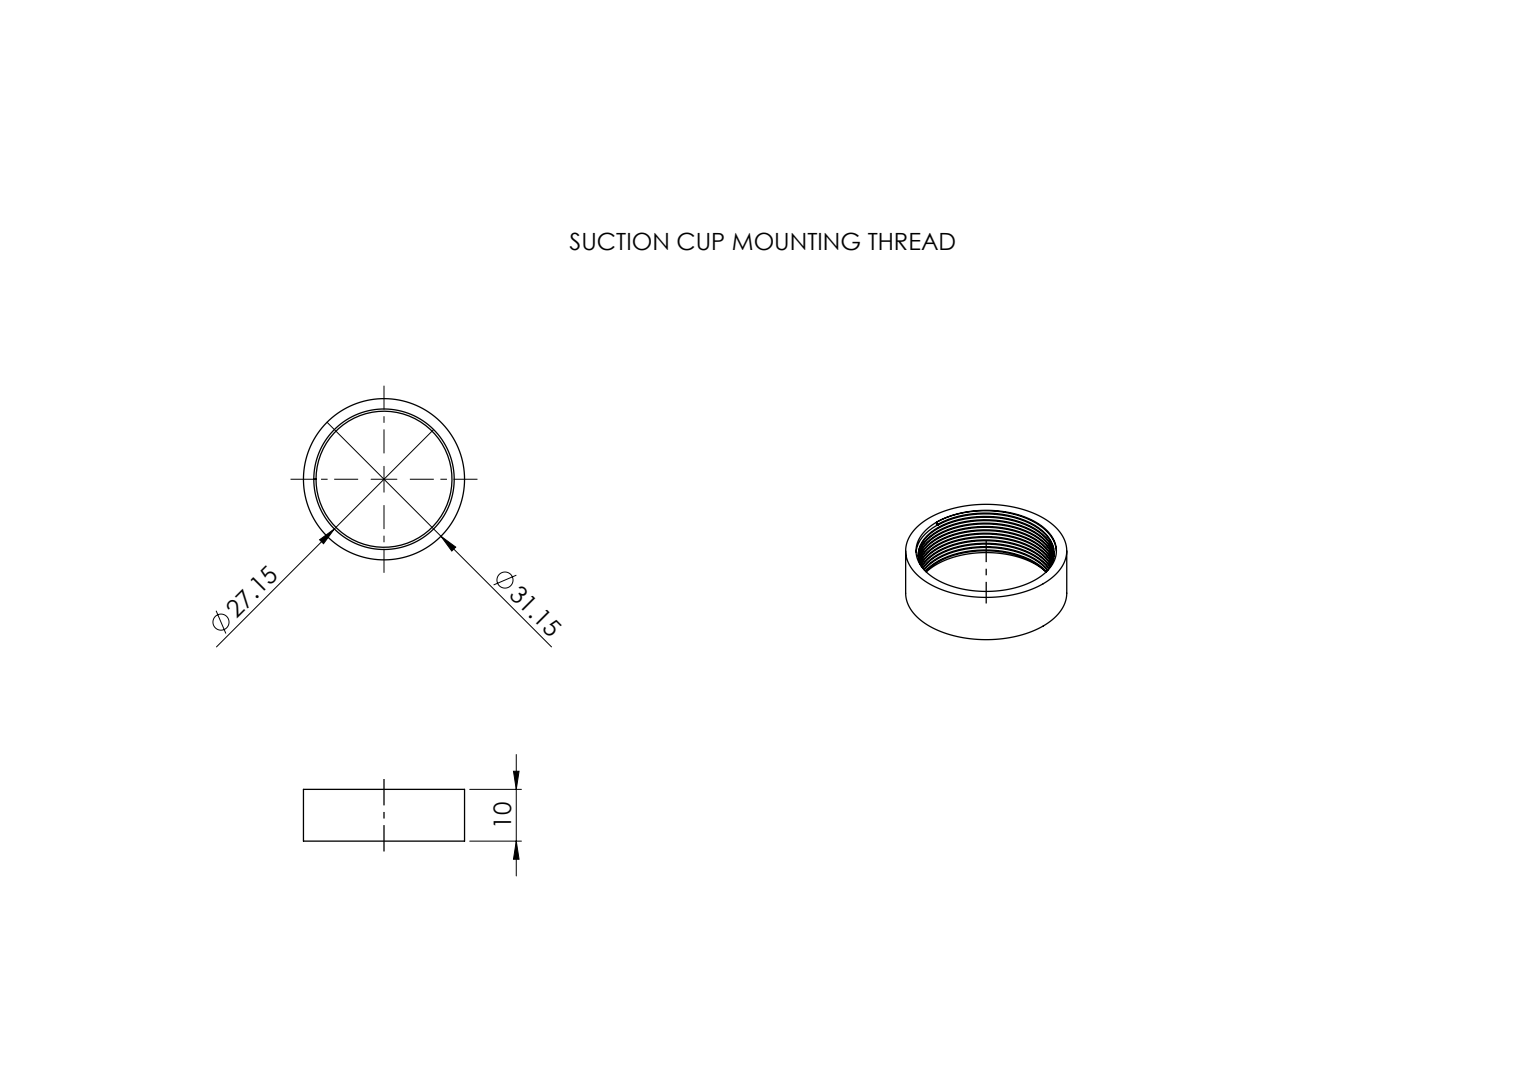
ISO-10303-21;
HEADER;
FILE_DESCRIPTION (('STEP AP214'),
    '1' );
FILE_NAME ('suction cup mounting thread.step',
    '2026-10-01T14:18:43',
    ( '' ),
    ( '' ),
    'SwSTEP 2.0',
    'SolidWorks 2026',
    '' );
FILE_SCHEMA (( 'AUTOMOTIVE_DESIGN' ));
ENDSEC;

DATA;
#15=CARTESIAN_POINT ( 'NONE',  ( 5.444914386472302859, 36.83281250108392868, 13.14518615778179189 ) ) ;
#34=VERTEX_POINT ( 'NONE', #6384 ) ;
#42=CARTESIAN_POINT ( 'NONE',  ( -13.36000105192242060, 40.87597656304196647, 0.000000000000000000 ) ) ;
#58=VERTEX_POINT ( 'NONE', #14643 ) ;
#60=CARTESIAN_POINT ( 'NONE',  ( -13.14518615778179900, 39.11484375108394573, -5.444914386472297529 ) ) ;
#65=CARTESIAN_POINT ( 'NONE',  ( -8.049105076161786076E-16, 38.96601562608393721, -13.14518615778179544 ) ) ;
#68=CARTESIAN_POINT ( 'NONE',  ( 2.493653234604083739E-15, 38.02343749999999289, 13.57481594606304576 ) ) ;
#72=CARTESIAN_POINT ( 'NONE',  ( 13.57481594606304931, 38.17226562499999432, 5.622872871577869525 ) ) ;
#73=CARTESIAN_POINT ( 'NONE',  ( 5.444914386472297529, 37.92421875108392726, -13.14518615778179900 ) ) ;
#89=CARTESIAN_POINT ( 'NONE',  ( -5.622872871577804688, 36.48554687716787726, 13.57481594606311504 ) ) ;
#92=ORIENTED_EDGE ( 'NONE', *, *, #1447, .F. ) ;
#108=CARTESIAN_POINT ( 'NONE',  ( 9.295050272127046043, 38.07304687608393579, -9.295050272127046043 ) ) ;
#109=CARTESIAN_POINT ( 'NONE',  ( -5.622872871577873077, 36.18789062716787441, -13.57481594606304753 ) ) ;
#127=CARTESIAN_POINT ( 'NONE',  ( 5.444914386472302859, 36.03906250108394005, 13.14518615778179189 ) ) ;
#138=VERTEX_POINT ( 'NONE', #3105 ) ;
#143=CARTESIAN_POINT ( 'NONE',  ( 9.598844408820456309, 34.35234374999999574, -9.598844408820458085 ) ) ;
#158=CARTESIAN_POINT ( 'NONE',  ( -9.295050272127046043, 36.48554687608393721, -9.295050272127046043 ) ) ;
#199=CARTESIAN_POINT ( 'NONE',  ( -13.14518615778179544, 37.57695312608393579, 0.000000000000000000 ) ) ;
#204=CARTESIAN_POINT ( 'NONE',  ( -9.295050272127046043, 36.68398437608393436, -9.295050272127046043 ) ) ;
#205=ADVANCED_FACE ( 'NONE', ( #10326 ), #4081, .F. ) ;
#211=CARTESIAN_POINT ( 'NONE',  ( -8.312177448680279460E-16, 36.83281249999999574, -13.57481594606304576 ) ) ;
#212=CARTESIAN_POINT ( 'NONE',  ( -13.14518615778179900, 38.12265625108393152, -5.444914386472297529 ) ) ;
#240=FACE_OUTER_BOUND ( 'NONE', #19523, .T. ) ;
#242=CARTESIAN_POINT ( 'NONE',  ( 1.662435489736055892E-15, 40.99999999999999289, 13.57481594606304576 ) ) ;
#247=CARTESIAN_POINT ( 'NONE',  ( 9.295050272127046043, 35.69179687608394147, -9.295050272127046043 ) ) ;
#248=CARTESIAN_POINT ( 'NONE',  ( 2.493653234604083739E-15, 37.32890625216786873, 13.57481594606304576 ) ) ;
#261=CARTESIAN_POINT ( 'NONE',  ( 1.662435489736055892E-15, 40.99999999999999289, 13.57481594606304576 ) ) ;
#263=ORIENTED_EDGE ( 'NONE', *, *, #18368, .T. ) ;
#269=CARTESIAN_POINT ( 'NONE',  ( -13.14518615778179189, 36.63437500108393152, 5.444914386472304635 ) ) ;
#300=CARTESIAN_POINT ( 'NONE',  ( 13.14518615778179544, 37.77539062608393294, -1.609821015232357215E-15 ) ) ;
#343=CARTESIAN_POINT ( 'NONE',  ( 2.414731522848535132E-15, 40.15664062608393436, 13.14518615778179544 ) ) ;
#349=CARTESIAN_POINT ( 'NONE',  ( 9.295050272127046043, 37.27929687608394005, -9.295050272127046043 ) ) ;
#355=CARTESIAN_POINT ( 'NONE',  ( 5.622872871577878406, 37.27929687499999289, 13.57481594606304576 ) ) ;
#356=CARTESIAN_POINT ( 'NONE',  ( -5.444914386472299306, 38.32109375108394289, 13.14518615778179722 ) ) ;
#367=PLANE ( 'NONE',  #22670 ) ;
#371=CARTESIAN_POINT ( 'NONE',  ( 0.000000000000000000, 40.99999999999999289, 0.000000000000000000 ) ) ;
#394=CARTESIAN_POINT ( 'NONE',  ( 5.444914386472297529, 38.12265625108393152, -13.14518615778179900 ) ) ;
#395=CARTESIAN_POINT ( 'NONE',  ( -9.598844408820454532, 37.22968750216787726, 9.598844408820459861 ) ) ;
#406=FACE_OUTER_BOUND ( 'NONE', #21933, .T. ) ;
#407=CARTESIAN_POINT ( 'NONE',  ( -8.312177448680279460E-16, 34.55078125216787299, -13.57481594606304576 ) ) ;
#414=CARTESIAN_POINT ( 'NONE',  ( -13.14518615778179189, 35.84062500108394289, 5.444914386472304635 ) ) ;
#416=CARTESIAN_POINT ( 'NONE',  ( 9.598844408820456309, 39.11484374999999858, -9.598844408820458085 ) ) ;
#441=CARTESIAN_POINT ( 'NONE',  ( 13.14518615778179544, 33.01289062608393010, -1.609821015232357215E-15 ) ) ;
#460=ADVANCED_FACE ( 'NONE', ( #11167, #24165 ), #367, .F. ) ;
#470=EDGE_CURVE ( 'NONE', #4431, #13527, #13159, .T. ) ;
#488=CARTESIAN_POINT ( 'NONE',  ( -9.295050272127046043, 35.09648437608393579, -9.295050272127046043 ) ) ;
#495=CARTESIAN_POINT ( 'NONE',  ( 13.14518615778179544, 36.38632812608393863, -1.609821015232357215E-15 ) ) ;
#500=CARTESIAN_POINT ( 'NONE',  ( 2.493653234604083739E-15, 33.26093749999999716, 13.57481594606304576 ) ) ;
#501=CARTESIAN_POINT ( 'NONE',  ( -8.049105076161786076E-16, 33.21132812608393436, -13.14518615778179544 ) ) ;
#535=CARTESIAN_POINT ( 'NONE',  ( -5.444914386472297529, 35.84062500108394289, -13.14518615778179900 ) ) ;
#536=CARTESIAN_POINT ( 'NONE',  ( -13.57481594606304576, 37.92421875216787441, 0.000000000000000000 ) ) ;
#548=CARTESIAN_POINT ( 'NONE',  ( -9.598844408820454532, 31.67343750216787512, 9.598844408820459861 ) ) ;
#557=CARTESIAN_POINT ( 'NONE',  ( -13.14518615778179900, 37.32890625108393579, -5.444914386472297529 ) ) ;
#586=CARTESIAN_POINT ( 'NONE',  ( -5.444914386472299306, 31.97109375108393792, 13.14518615778179722 ) ) ;
#617=AXIS2_PLACEMENT_3D ( 'NONE', #8449, #19290, #20876 ) ;
#629=CARTESIAN_POINT ( 'NONE',  ( 13.14518615778179900, 36.33671875108394289, 5.444914386472293977 ) ) ;
#636=CARTESIAN_POINT ( 'NONE',  ( -13.14518615778179189, 39.21406250108392300, 5.444914386472304635 ) ) ;
#637=VERTEX_POINT ( 'NONE', #2015 ) ;
#643=CARTESIAN_POINT ( 'NONE',  ( 5.622872871577878406, 33.31054687499999289, 13.57481594606304576 ) ) ;
#644=CARTESIAN_POINT ( 'NONE',  ( 5.444914386472297529, 33.16171875108393152, -13.14518615778179900 ) ) ;
#661=( NAMED_UNIT ( * ) SI_UNIT ( $, .STERADIAN. ) SOLID_ANGLE_UNIT ( ) );
#680=CARTESIAN_POINT ( 'NONE',  ( 13.14518615778179900, 33.95546875108393436, 5.444914386472293977 ) ) ;
#681=CARTESIAN_POINT ( 'NONE',  ( -13.57481594606304576, 33.95546875216787441, 0.000000000000000000 ) ) ;
#695=CARTESIAN_POINT ( 'NONE',  ( 0.000000000000000000, 40.99999999999999289, -13.57481594606304576 ) ) ;
#701=CARTESIAN_POINT ( 'NONE',  ( 13.14518615778179900, 34.65000000108393152, -5.444914386472297529 ) ) ;
#717=CARTESIAN_POINT ( 'NONE',  ( -8.312177448680279460E-16, 34.45156249999999432, -13.57481594606304576 ) ) ;
#729=CARTESIAN_POINT ( 'NONE',  ( -5.444914386472297529, 32.46718750108393436, -13.14518615778179722 ) ) ;
#772=CARTESIAN_POINT ( 'NONE',  ( -5.444914386472297529, 36.63437500108393152, -13.14518615778179900 ) ) ;
#779=CARTESIAN_POINT ( 'NONE',  ( -8.049105076161786076E-16, 34.99726562608393721, -13.14518615778179544 ) ) ;
#787=CARTESIAN_POINT ( 'NONE',  ( -8.312177448680279460E-16, 32.86406249999999574, -13.57481594606304576 ) ) ;
#788=CARTESIAN_POINT ( 'NONE',  ( 9.295050272127047819, 35.29492187608393294, 9.295050272127046043 ) ) ;
#797=CARTESIAN_POINT ( 'NONE',  ( 7.171391216998964424, 31.99955315621561525, -11.52591757658528948 ) ) ;
#806=SURFACE_STYLE_USAGE ( .BOTH. , #11458 ) ;
#824=ADVANCED_FACE ( 'NONE', ( #21683 ), #14677, .F. ) ;
#827=CARTESIAN_POINT ( 'NONE',  ( -5.444914386472297529, 32.66562500108393863, -13.14518615778179900 ) ) ;
#828=CARTESIAN_POINT ( 'NONE',  ( 13.57481594606304753, 35.19570312716788152, -5.622872871577873077 ) ) ;
#839=DIRECTION ( 'NONE',  ( -0.000000000000000000, -1.000000000000000000, -0.000000000000000000 ) ) ;
#846=CARTESIAN_POINT ( 'NONE',  ( -5.622872871577828668, 33.21132812499999432, 13.57481594606309194 ) ) ;
#848=CARTESIAN_POINT ( 'NONE',  ( 13.14518615778179544, 32.21914062608393436, -1.609821015232357215E-15 ) ) ;
#852=CARTESIAN_POINT ( 'NONE',  ( -8.312177448680279460E-16, 37.72578125216787726, -13.57481594606304576 ) ) ;
#859=CARTESIAN_POINT ( 'NONE',  ( -8.312177448680279460E-16, 38.51953125216787299, -13.57481594606304576 ) ) ;
#862=DIRECTION ( 'NONE',  ( -0.000000000000000000, -1.000000000000000000, -0.000000000000000000 ) ) ;
#878=CARTESIAN_POINT ( 'NONE',  ( -5.444914386472297529, 33.26093750108393721, -13.14518615778179722 ) ) ;
#891=VECTOR ( 'NONE', #4255, 1000.000000000000000 ) ;
#917=CARTESIAN_POINT ( 'NONE',  ( -8.049105076161786076E-16, 37.37851562608393863, -13.14518615778179544 ) ) ;
#924=CARTESIAN_POINT ( 'NONE',  ( -8.049105076161786076E-16, 33.40976562608393863, -13.14518615778179544 ) ) ;
#930=EDGE_CURVE ( 'NONE', #20608, #21855, #13534, .T. ) ;
#931=CARTESIAN_POINT ( 'NONE',  ( -9.598844408820458085, 32.96328124999999432, -9.598844408820458085 ) ) ;
#932=CARTESIAN_POINT ( 'NONE',  ( -8.049105076161786076E-16, 32.41757812608393863, -13.14518615778179544 ) ) ;
#937=ORIENTED_EDGE ( 'NONE', *, *, #26334, .F. ) ;
#944=CARTESIAN_POINT ( 'NONE',  ( 5.622872871578054266, 32.11992187716787583, -13.57481594606286635 ) ) ;
#947=VERTEX_POINT ( 'NONE', #24667 ) ;
#952=CYLINDRICAL_SURFACE ( 'NONE', #25355, 13.57481594606304576 ) ;
#967=CARTESIAN_POINT ( 'NONE',  ( -13.14518615778179544, 33.60820312608393579, 0.000000000000000000 ) ) ;
#968=CARTESIAN_POINT ( 'NONE',  ( 13.57481594606304753, 34.40195312716787157, -5.622872871577873077 ) ) ;
#975=CARTESIAN_POINT ( 'NONE',  ( 2.493653234604083739E-15, 37.32890625216786873, 13.57481594606304576 ) ) ;
#989=CARTESIAN_POINT ( 'NONE',  ( -13.57481594606304576, 33.06249999999999289, 0.000000000000000000 ) ) ;
#991=CARTESIAN_POINT ( 'NONE',  ( -8.049105076161786076E-16, 34.00507812608393721, -13.14518615778179544 ) ) ;
#994=CARTESIAN_POINT ( 'NONE',  ( 13.57481594606304576, 37.52734375216787299, -1.662435489736055892E-15 ) ) ;
#995=CARTESIAN_POINT ( 'NONE',  ( -13.57481594606304576, 35.44374999999999432, 0.000000000000000000 ) ) ;
#1021=CARTESIAN_POINT ( 'NONE',  ( 9.295050272127046043, 32.31835937608393294, -9.295050272127046043 ) ) ;
#1046=ORIENTED_EDGE ( 'NONE', *, *, #15737, .F. ) ;
#1060=CARTESIAN_POINT ( 'NONE',  ( 5.444914386472297529, 35.74140625108393721, -13.14518615778179900 ) ) ;
#1067=CARTESIAN_POINT ( 'NONE',  ( 9.295050272127046043, 35.69179687608394147, -9.295050272127046043 ) ) ;
#1069=CARTESIAN_POINT ( 'NONE',  ( 2.493653234604083739E-15, 36.43593749999999432, 13.57481594606304576 ) ) ;
#1072=CARTESIAN_POINT ( 'NONE',  ( -13.57481594606304576, 32.26874999999999716, 0.000000000000000000 ) ) ;
#1073=CARTESIAN_POINT ( 'NONE',  ( 13.14518615778179900, 34.65000000108393152, -5.444914386472297529 ) ) ;
#1109=CARTESIAN_POINT ( 'NONE',  ( -9.295050272127046043, 33.50898437608393010, -9.295050272127046043 ) ) ;
#1110=CARTESIAN_POINT ( 'NONE',  ( 2.493653234604083739E-15, 35.74140625216787015, 13.57481594606304576 ) ) ;
#1119=EDGE_LOOP ( 'NONE', ( #16453, #20874 ) ) ;
#1129=CARTESIAN_POINT ( 'NONE',  ( 13.57481594606304753, 40.65273437499999432, -5.622872871577873966 ) ) ;
#1131=CARTESIAN_POINT ( 'NONE',  ( 13.14518615778179544, 33.80664062608393294, -1.609821015232357215E-15 ) ) ;
#1135=CARTESIAN_POINT ( 'NONE',  ( 5.622872871577786924, 37.37851562716787157, 13.57481594606313813 ) ) ;
#1171=CARTESIAN_POINT ( 'NONE',  ( 9.598844408820459861, 35.84062500216786873, 9.598844408820456309 ) ) ;
#1201=CARTESIAN_POINT ( 'NONE',  ( 9.295050272127046043, 33.31054687608394005, -9.295050272127046043 ) ) ;
#1209=CARTESIAN_POINT ( 'NONE',  ( 2.414731522848535132E-15, 36.18789062608393436, 13.14518615778179544 ) ) ;
#1225=CARTESIAN_POINT ( 'NONE',  ( -5.622872871577873966, 33.70742187499999432, -13.57481594606304753 ) ) ;
#1231=ORIENTED_EDGE ( 'NONE', *, *, #22053, .F. ) ;
#1245=CARTESIAN_POINT ( 'NONE',  ( 2.414731522848535132E-15, 32.21914062608393436, 13.14518615778179544 ) ) ;
#1246=CARTESIAN_POINT ( 'NONE',  ( -5.622872871577873077, 33.31054687716787299, 13.57481594606304753 ) ) ;
#1265=LINE ( 'NONE', #3115, #23908 ) ;
#1267=CARTESIAN_POINT ( 'NONE',  ( -13.14518615778179544, 34.20351562608393436, 0.000000000000000000 ) ) ;
#1308=CARTESIAN_POINT ( 'NONE',  ( 0.000000000000000000, 40.99999999999999289, 0.000000000000000000 ) ) ;
#1310=AXIS2_PLACEMENT_3D ( 'NONE', #21064, #21343, #23065 ) ;
#1313=EDGE_CURVE ( 'NONE', #21025, #17571, #11932, .T. ) ;
#1317=ORIENTED_EDGE ( 'NONE', *, *, #20419, .T. ) ;
#1326=CARTESIAN_POINT ( 'NONE',  ( -5.444914386472297529, 39.61093750108393152, -13.14518615778179722 ) ) ;
#1337=CARTESIAN_POINT ( 'NONE',  ( 6.944426393311538881, 31.75150625057403175, -11.16113171639042356 ) ) ;
#1344=CARTESIAN_POINT ( 'NONE',  ( -5.444914386472297529, 35.04687500108393294, -13.14518615778179722 ) ) ;
#1355=ORIENTED_EDGE ( 'NONE', *, *, #12984, .F. ) ;
#1377=DIRECTION ( 'NONE',  ( 0.000000000000000000, 1.000000000000000000, 0.000000000000000000 ) ) ;
#1385=CARTESIAN_POINT ( 'NONE',  ( -13.57481594606304753, 40.15664062500000142, -5.622872871577873077 ) ) ;
#1386=CARTESIAN_POINT ( 'NONE',  ( -13.57481594606304753, 32.31835937716786589, -5.622872871577873077 ) ) ;
#1403=CARTESIAN_POINT ( 'NONE',  ( 0.000000000000000000, 40.99999999999999289, -13.57481594606304576 ) ) ;
#1406=EDGE_LOOP ( 'NONE', ( #23949, #8331, #11999, #3725 ) ) ;
#1447=EDGE_CURVE ( 'NONE', #17326, #28027, #2482, .T. ) ;
#1466=CARTESIAN_POINT ( 'NONE',  ( -5.444914386472297529, 38.02343750108394005, -13.14518615778179722 ) ) ;
#1474=CARTESIAN_POINT ( 'NONE',  ( 2.414731522848535132E-15, 33.80664062608393294, 13.14518615778179544 ) ) ;
#1494=VERTEX_POINT ( 'NONE', #14891 ) ;
#1503=DIRECTION ( 'NONE',  ( -0.8490667072653959035, 1.618318251311064231E-06, -0.5282856486891157610 ) ) ;
#1513=CARTESIAN_POINT ( 'NONE',  ( 9.295050272127047819, 40.25585937608393294, 9.295050272127046043 ) ) ;
#1519=AXIS2_PLACEMENT_3D ( 'NONE', #14564, #16851, #14693 ) ;
#1522=CARTESIAN_POINT ( 'NONE',  ( 5.622872871577871301, 38.37070312499999147, -13.57481594606304753 ) ) ;
#1523=CARTESIAN_POINT ( 'NONE',  ( 2.493653234604083739E-15, 32.56640625216787299, 13.57481594606304576 ) ) ;
#1532=FACE_OUTER_BOUND ( 'NONE', #20108, .T. ) ;
#1541=AXIS2_PLACEMENT_3D ( 'NONE', #2821, #839, #9509 ) ;
#1564=CARTESIAN_POINT ( 'NONE',  ( 9.295050272127046043, 39.66054687608393436, -9.295050272127046043 ) ) ;
#1605=CARTESIAN_POINT ( 'NONE',  ( 9.295050272127046043, 37.87460937608393152, -9.295050272127046043 ) ) ;
#1609=ORIENTED_EDGE ( 'NONE', *, *, #12107, .F. ) ;
#1614=CARTESIAN_POINT ( 'NONE',  ( 9.295050272127046043, 34.10429687608393579, -9.295050272127046043 ) ) ;
#1621=CARTESIAN_POINT ( 'NONE',  ( 13.14518615778179544, 32.41757812608393863, -1.609821015232357215E-15 ) ) ;
#1627=CARTESIAN_POINT ( 'NONE',  ( -5.622872871577965448, 32.41757812499999858, 13.57481594606295161 ) ) ;
#1640=CARTESIAN_POINT ( 'NONE',  ( 9.598844408820459861, 31.87187500216787228, 9.598844408820456309 ) ) ;
#1654=CARTESIAN_POINT ( 'NONE',  ( 5.622872871577878406, 39.66054687500000142, 13.57481594606304576 ) ) ;
#1655=CARTESIAN_POINT ( 'NONE',  ( -5.444914386472297529, 40.40468750108393436, -13.14518615778179900 ) ) ;
#1690=APPLICATION_CONTEXT ( 'automotive_design' ) ;
#1698=CARTESIAN_POINT ( 'NONE',  ( 13.14518615778179900, 40.40468750108393436, -5.444914386472297529 ) ) ;
#1716=CARTESIAN_POINT ( 'NONE',  ( -5.444914386472299306, 39.11484375108394573, 13.14518615778179722 ) ) ;
#1722=DIRECTION ( 'NONE',  ( 1.374060148949977908E-06, 0.9999999999986906030, 8.549343071804204525E-07 ) ) ;
#1734=ORIENTED_EDGE ( 'NONE', *, *, #1871, .F. ) ;
#1742=CARTESIAN_POINT ( 'NONE',  ( -5.444914386472297529, 38.81718750108393579, -13.14518615778179722 ) ) ;
#1753=CARTESIAN_POINT ( 'NONE',  ( 13.14518615778179544, 32.41757812608393863, -1.609821015232357215E-15 ) ) ;
#1783=CARTESIAN_POINT ( 'NONE',  ( -8.049105076161786076E-16, 33.21132812608393436, -13.14518615778179544 ) ) ;
#1796=CARTESIAN_POINT ( 'NONE',  ( -13.57481594606304753, 40.95039062499999005, -5.622872871577873077 ) ) ;
#1797=CARTESIAN_POINT ( 'NONE',  ( 5.444914386472302859, 39.21406250108392300, 13.14518615778179189 ) ) ;
#1809=CARTESIAN_POINT ( 'NONE',  ( -5.622872871577873966, 34.79882812499999289, 13.57481594606304753 ) ) ;
#1816=ORIENTED_EDGE ( 'NONE', *, *, #14513, .T. ) ;
#1838=CARTESIAN_POINT ( 'NONE',  ( -9.598844408820458085, 40.20625000216787726, -9.598844408820458085 ) ) ;
#1854=CARTESIAN_POINT ( 'NONE',  ( -5.444914386472297529, 38.02343750108394005, -13.14518615778179900 ) ) ;
#1871=EDGE_CURVE ( 'NONE', #9928, #16597, #27628, .T. ) ;
#1876=CARTESIAN_POINT ( 'NONE',  ( -13.57481594606304398, 33.21132812716787441, 5.622872871577880183 ) ) ;
#1879=ORIENTED_EDGE ( 'NONE', *, *, #9511, .T. ) ;
#1883=CARTESIAN_POINT ( 'NONE',  ( 5.444914386472302859, 39.21406250108392300, 13.14518615778179189 ) ) ;
#1906=CARTESIAN_POINT ( 'NONE',  ( -13.57481594606304576, 37.13046875216787868, 0.000000000000000000 ) ) ;
#1911=DIRECTION ( 'NONE',  ( 1.000000000000000000, 0.000000000000000000, -0.000000000000000000 ) ) ;
#1912=CARTESIAN_POINT ( 'NONE',  ( 0.000000000000000000, 40.99999999999999289, 0.000000000000000000 ) ) ;
#1919=CYLINDRICAL_SURFACE ( 'NONE', #9601, 13.57481594606304576 ) ;
#1923=CARTESIAN_POINT ( 'NONE',  ( 5.444914386472302859, 38.61875000108393152, 13.14518615778179189 ) ) ;
#1928=CARTESIAN_POINT ( 'NONE',  ( 2.414731522848535132E-15, 40.15664062608393436, 13.14518615778179544 ) ) ;
#1934=CARTESIAN_POINT ( 'NONE',  ( -5.622872871577873077, 39.26367187499999289, -13.57481594606304753 ) ) ;
#1935=CARTESIAN_POINT ( 'NONE',  ( 5.444914386472297529, 40.30546875108393579, -13.14518615778179900 ) ) ;
#1949=( LENGTH_UNIT ( ) NAMED_UNIT ( * ) SI_UNIT ( .MILLI., .METRE. ) );
#1968=ORIENTED_EDGE ( 'NONE', *, *, #8452, .F. ) ;
#1970=CARTESIAN_POINT ( 'NONE',  ( 13.14518615778179900, 38.81718750108393579, -5.444914386472297529 ) ) ;
#1989=CARTESIAN_POINT ( 'NONE',  ( -13.14518615778179900, 38.12265625108393152, -5.444914386472297529 ) ) ;
#2000=VERTEX_POINT ( 'NONE', #4164 ) ;
#2006=EDGE_LOOP ( 'NONE', ( #20300, #6817, #20484, #23254 ) ) ;
#2014=CARTESIAN_POINT ( 'NONE',  ( 13.14518615778179544, 36.18789062608393436, -1.609821015232357215E-15 ) ) ;
#2015=CARTESIAN_POINT ( 'NONE',  ( 1.662435489736055892E-15, 40.99999999999999289, 13.57481594606304576 ) ) ;
#2021=DIRECTION ( 'NONE',  ( -0.000000000000000000, -1.000000000000000000, -0.000000000000000000 ) ) ;
#2029=CARTESIAN_POINT ( 'NONE',  ( 1.662435489736055892E-15, 40.99999999999999289, 13.57481594606304576 ) ) ;
#2058=CARTESIAN_POINT ( 'NONE',  ( 9.295050272127046043, 38.07304687608393579, -9.295050272127046043 ) ) ;
#2063=CARTESIAN_POINT ( 'NONE',  ( 13.14518615778179722, 40.40468750108393436, -5.444914386472297529 ) ) ;
#2065=CARTESIAN_POINT ( 'NONE',  ( -13.57481594606304753, 37.77539062499998579, -5.622872871577872189 ) ) ;
#2069=CARTESIAN_POINT ( 'NONE',  ( -5.622872871577873077, 36.88242187499999858, -13.57481594606304753 ) ) ;
#2070=CARTESIAN_POINT ( 'NONE',  ( -5.444914386472299306, 35.93984375108392726, 13.14518615778179722 ) ) ;
#2077=ORIENTED_EDGE ( 'NONE', *, *, #19944, .F. ) ;
#2089=VECTOR ( 'NONE', #21736, 1000.000000000000000 ) ;
#2101=CARTESIAN_POINT ( 'NONE',  ( -13.57481594606304753, 39.36289062499999858, -5.622872871577872189 ) ) ;
#2102=CARTESIAN_POINT ( 'NONE',  ( -8.312177448680279460E-16, 37.62656249999999858, -13.57481594606304576 ) ) ;
#2108=CARTESIAN_POINT ( 'NONE',  ( -13.14518615778179544, 38.37070312608393152, 0.000000000000000000 ) ) ;
#2109=CARTESIAN_POINT ( 'NONE',  ( -13.57481594606304753, 36.28710937716787299, -5.622872871577873077 ) ) ;
#2116=VERTEX_POINT ( 'NONE', #21973 ) ;
#2128=CARTESIAN_POINT ( 'NONE',  ( 9.295050272127047819, 40.05742187608392868, 9.295050272127046043 ) ) ;
#2157=( BOUNDED_CURVE ( )  B_SPLINE_CURVE ( 2, ( #26013, #4216, #6076, #14743, #12873, #4080, #6345, #13012, #10612 ),
 .UNSPECIFIED., .F., .F. ) 
 B_SPLINE_CURVE_WITH_KNOTS ( ( 3, 2, 2, 2, 3 ),
 ( 0.1458333333333336757, 0.1562500000000002776, 0.1666666666666669072, 0.1770833333333335369, 0.1875000000000001388 ),
 .UNSPECIFIED. ) 
 CURVE ( )  GEOMETRIC_REPRESENTATION_ITEM ( )  RATIONAL_B_SPLINE_CURVE ( ( 0.9999999999999975575, 0.9238795325112891810, 1.000000000000000000, 0.9238795325112867385, 1.000000000000000000, 0.9238795325112867385, 1.000000000000000000, 0.9238795325112857393, 1.000000000000001110 ) ) 
 REPRESENTATION_ITEM ( '' )  );
#2158=CARTESIAN_POINT ( 'NONE',  ( 13.14518615778179722, 35.34453125108392157, 5.444914386472293977 ) ) ;
#2164=FACE_OUTER_BOUND ( 'NONE', #18756, .T. ) ;
#2202=CARTESIAN_POINT ( 'NONE',  ( -8.049105076161786076E-16, 40.55351562608393579, -13.14518615778179544 ) ) ;
#2208=CARTESIAN_POINT ( 'NONE',  ( 13.14518615778179722, 39.51171875108393294, 5.444914386472293977 ) ) ;
#2209=CARTESIAN_POINT ( 'NONE',  ( -5.622872871577890841, 39.66054687716787441, 13.57481594606302444 ) ) ;
#2213=AXIS2_PLACEMENT_3D ( 'NONE', #10774, #17198, #4241 ) ;
#2216=CARTESIAN_POINT ( 'NONE',  ( -13.57481594606304576, 37.03124999999999289, 0.000000000000000000 ) ) ;
#2217=CARTESIAN_POINT ( 'NONE',  ( -13.14518615778179189, 35.84062500108394289, 5.444914386472304635 ) ) ;
#2231=CARTESIAN_POINT ( 'NONE',  ( -9.598844408820454532, 34.74921874999999716, 9.598844408820459861 ) ) ;
#2233=VECTOR ( 'NONE', #26227, 1000.000000000000000 ) ;
#2247=B_SPLINE_CURVE_WITH_KNOTS ( 'NONE', 3,
 ( #26875, #18454, #5344, #2915 ),
 .UNSPECIFIED., .F., .F.,
 ( 4, 4 ),
 ( 0.000000000000000000, 1.000000000000000000 ),
 .UNSPECIFIED. ) ;
#2248=CYLINDRICAL_SURFACE ( 'NONE', #9842, 13.57481594606304576 ) ;
#2250=DIRECTION ( 'NONE',  ( -0.000000000000000000, -1.000000000000000000, -0.000000000000000000 ) ) ;
#2254=CARTESIAN_POINT ( 'NONE',  ( -8.312177448680279460E-16, 34.55078125216787299, -13.57481594606304576 ) ) ;
#2255=CARTESIAN_POINT ( 'NONE',  ( -13.14518615778179544, 37.57695312608393579, 0.000000000000000000 ) ) ;
#2256=CARTESIAN_POINT ( 'NONE',  ( -5.622872871577873077, 37.27929687716787299, 13.57481594606304753 ) ) ;
#2273=CARTESIAN_POINT ( 'NONE',  ( 0.000000000000000000, 40.99999999999999289, -15.57481594606304576 ) ) ;
#2275=CARTESIAN_POINT ( 'NONE',  ( 2.414731522848535132E-15, 39.16445312608392726, 13.14518615778179544 ) ) ;
#2278=DIRECTION ( 'NONE',  ( 0.000000000000000000, 0.000000000000000000, -1.000000000000000000 ) ) ;
#2291=CARTESIAN_POINT ( 'NONE',  ( 13.57481594606304931, 34.20351562499999432, 5.622872871577868636 ) ) ;
#2302=CARTESIAN_POINT ( 'NONE',  ( 5.444914386472297529, 37.13046875108393152, -13.14518615778179722 ) ) ;
#2311=CARTESIAN_POINT ( 'NONE',  ( 0.000000000000000000, 40.99999999999999289, 0.000000000000000000 ) ) ;
#2315=LINE ( 'NONE', #15103, #16400 ) ;
#2316=DIRECTION ( 'NONE',  ( -0.000000000000000000, -1.000000000000000000, -0.000000000000000000 ) ) ;
#2317=FACE_OUTER_BOUND ( 'NONE', #13417, .T. ) ;
#2339=CARTESIAN_POINT ( 'NONE',  ( 0.000000000000000000, 40.99999999999999289, 0.000000000000000000 ) ) ;
#2345=CARTESIAN_POINT ( 'NONE',  ( -13.14518615778179900, 38.32109375108394289, -5.444914386472297529 ) ) ;
#2351=CARTESIAN_POINT ( 'NONE',  ( -9.295050272127044266, 38.46992187608393721, 9.295050272127047819 ) ) ;
#2358=CARTESIAN_POINT ( 'NONE',  ( -9.598844408820458085, 35.34453124999998863, -9.598844408820458085 ) ) ;
#2359=CARTESIAN_POINT ( 'NONE',  ( 5.444914386472302859, 36.03906250108394005, 13.14518615778179189 ) ) ;
#2372=CARTESIAN_POINT ( 'NONE',  ( -9.598844408820458085, 34.55078124999999289, -9.598844408820458085 ) ) ;
#2373=EDGE_CURVE ( 'NONE', #2719, #1494, #18964, .T. ) ;
#2396=CARTESIAN_POINT ( 'NONE',  ( -9.295050272127046043, 38.27148437608393294, -9.295050272127046043 ) ) ;
#2397=CARTESIAN_POINT ( 'NONE',  ( -8.312177448680279460E-16, 38.51953125216787299, -13.57481594606304576 ) ) ;
#2416=CARTESIAN_POINT ( 'NONE',  ( -5.444914386472299306, 35.14609375108393152, 13.14518615778179722 ) ) ;
#2442=CARTESIAN_POINT ( 'NONE',  ( 9.295050272127046043, 37.08085937608393579, -9.295050272127046043 ) ) ;
#2460=CARTESIAN_POINT ( 'NONE',  ( 0.000000000000000000, 40.99999999999999289, -13.57481594606304576 ) ) ;
#2469=CARTESIAN_POINT ( 'NONE',  ( 13.57481594606304576, 33.55859375216787299, -1.662435489736055892E-15 ) ) ;
#2475=CARTESIAN_POINT ( 'NONE',  ( 13.57481594606304576, 37.42812499999999432, -1.662435489736055892E-15 ) ) ;
#2479=CARTESIAN_POINT ( 'NONE',  ( -5.444914386472297529, 39.80937500108392868, -13.14518615778179900 ) ) ;
#2482=( BOUNDED_CURVE ( )  B_SPLINE_CURVE ( 2, ( #20922, #23059, #27618, #3809, #6224, #16771, #25328, #12469, #10336 ),
 .UNSPECIFIED., .F., .F. ) 
 B_SPLINE_CURVE_WITH_KNOTS ( ( 3, 2, 2, 2, 3 ),
 ( 0.8124999999999998890, 0.8229166666666666297, 0.8333333333333334814, 0.8437500000000003331, 0.8541666666666670737 ),
 .UNSPECIFIED. ) 
 CURVE ( )  GEOMETRIC_REPRESENTATION_ITEM ( )  RATIONAL_B_SPLINE_CURVE ( ( 1.000000000000000888, 0.9238795325112859613, 1.000000000000000000, 0.9238795325112867385, 1.000000000000000000, 0.9238795325112867385, 1.000000000000000000, 0.9238795325112835188, 1.000000000000003331 ) ) 
 REPRESENTATION_ITEM ( '' )  );
#2486=CARTESIAN_POINT ( 'NONE',  ( -13.14518615778179722, 38.32109375108394289, -5.444914386472297529 ) ) ;
#2493=CARTESIAN_POINT ( 'NONE',  ( -5.622872871577873077, 36.08867187500000284, -13.57481594606304753 ) ) ;
#2494=CARTESIAN_POINT ( 'NONE',  ( -8.049105076161786076E-16, 35.59257812608393579, -13.14518615778179544 ) ) ;
#2508=CARTESIAN_POINT ( 'NONE',  ( -13.57481594606304398, 36.38632812716788578, 5.622872871577880183 ) ) ;
#2517=DIRECTION ( 'NONE',  ( 0.000000000000000000, 1.000000000000000000, 0.000000000000000000 ) ) ;
#2523=CARTESIAN_POINT ( 'NONE',  ( -8.312177448680279460E-16, 39.21406249999999716, -13.57481594606304576 ) ) ;
#2530=CARTESIAN_POINT ( 'NONE',  ( -13.14518615778179189, 36.03906250108394005, 5.444914386472304635 ) ) ;
#2531=CARTESIAN_POINT ( 'NONE',  ( -5.622872871577873077, 37.77539062716788010, -13.57481594606304753 ) ) ;
#2548=CARTESIAN_POINT ( 'NONE',  ( 13.57481594606304576, 34.35234375216787583, -1.662435489736055892E-15 ) ) ;
#2553=DIRECTION ( 'NONE',  ( -0.000000000000000000, -1.000000000000000000, -0.000000000000000000 ) ) ;
#2555=CARTESIAN_POINT ( 'NONE',  ( 9.295050272127047819, 37.67617187608393436, 9.295050272127046043 ) ) ;
#2585=CARTESIAN_POINT ( 'NONE',  ( 5.444914386472297529, 35.54296875108393294, -13.14518615778179722 ) ) ;
#2607=ORIENTED_EDGE ( 'NONE', *, *, #18989, .F. ) ;
#2625=CARTESIAN_POINT ( 'NONE',  ( -13.14518615778179544, 35.19570312608393436, 0.000000000000000000 ) ) ;
#2632=CARTESIAN_POINT ( 'NONE',  ( 5.444914386472297529, 38.91640625108393436, -13.14518615778179722 ) ) ;
#2637=CARTESIAN_POINT ( 'NONE',  ( 13.57481594606304931, 37.37851562499999858, 5.622872871577869525 ) ) ;
#2638=CARTESIAN_POINT ( 'NONE',  ( 13.14518615778179900, 36.93203125108394147, 5.444914386472293977 ) ) ;
#2674=CARTESIAN_POINT ( 'NONE',  ( 13.14518615778179900, 37.22968750108393721, -5.444914386472297529 ) ) ;
#2675=CARTESIAN_POINT ( 'NONE',  ( 9.598844408820456309, 38.42031250216787441, -9.598844408820458085 ) ) ;
#2681=VECTOR ( 'NONE', #18208, 1000.000000000000000 ) ;
#2695=CARTESIAN_POINT ( 'NONE',  ( -8.049105076161786076E-16, 35.59257812608393579, -13.14518615778179544 ) ) ;
#2719=VERTEX_POINT ( 'NONE', #7023 ) ;
#2725=CARTESIAN_POINT ( 'NONE',  ( 13.14518615778179544, 34.60039062608392868, -1.609821015232357215E-15 ) ) ;
#2742=ORIENTED_EDGE ( 'NONE', *, *, #930, .F. ) ;
#2766=CARTESIAN_POINT ( 'NONE',  ( -9.295050272127046043, 35.89023437608393152, -9.295050272127046043 ) ) ;
#2772=CARTESIAN_POINT ( 'NONE',  ( -5.444914386472299306, 38.51953125108393294, 13.14518615778179722 ) ) ;
#2773=CARTESIAN_POINT ( 'NONE',  ( -8.312177448680279460E-16, 36.03906250000000000, -13.57481594606304576 ) ) ;
#2777=CARTESIAN_POINT ( 'NONE',  ( -9.598844408820458085, 32.16953124999999147, -9.598844408820458085 ) ) ;
#2778=CARTESIAN_POINT ( 'NONE',  ( -9.295050272127046043, 34.89804687608393152, -9.295050272127046043 ) ) ;
#2784=ORIENTED_EDGE ( 'NONE', *, *, #12107, .T. ) ;
#2790=CARTESIAN_POINT ( 'NONE',  ( 2.493653234604083739E-15, 36.43593749999999432, 13.57481594606304576 ) ) ;
#2809=CARTESIAN_POINT ( 'NONE',  ( -5.444914386472299306, 32.16953125108393152, 13.14518615778179722 ) ) ;
#2810=CARTESIAN_POINT ( 'NONE',  ( 9.598844408820456309, 35.24531250216787726, -9.598844408820458085 ) ) ;
#2821=CARTESIAN_POINT ( 'NONE',  ( 0.000000000000000000, 40.99999999999999289, 0.000000000000000000 ) ) ;
#2831=CARTESIAN_POINT ( 'NONE',  ( 9.295050272127046043, 34.69960937608393436, -9.295050272127046043 ) ) ;
#2834=CARTESIAN_POINT ( 'NONE',  ( -5.622872871577839327, 38.07304687716787583, 13.57481594606308128 ) ) ;
#2847=CARTESIAN_POINT ( 'NONE',  ( 9.598844408820459861, 34.15390624999999858, 9.598844408820456309 ) ) ;
#2858=CARTESIAN_POINT ( 'NONE',  ( -5.444914386472299306, 33.55859375108393294, 13.14518615778179722 ) ) ;
#2899=CARTESIAN_POINT ( 'NONE',  ( -13.14518615778179900, 36.73359375108393010, -5.444914386472297529 ) ) ;
#2905=CARTESIAN_POINT ( 'NONE',  ( 5.444914386472302859, 35.44375000108393436, 13.14518615778179189 ) ) ;
#2911=CARTESIAN_POINT ( 'NONE',  ( -5.622872871577873077, 34.79882812499998579, 13.57481594606304753 ) ) ;
#2912=CARTESIAN_POINT ( 'NONE',  ( -13.14518615778179544, 34.20351562608393436, 0.000000000000000000 ) ) ;
#2915=CARTESIAN_POINT ( 'NONE',  ( 7.171390501253594785, 31.30502191632583830, -11.52591802191987114 ) ) ;
#2917=EDGE_LOOP ( 'NONE', ( #4462, #19296, #4936, #14694 ) ) ;
#2924=CARTESIAN_POINT ( 'NONE',  ( -13.57481594606304753, 34.69960937716787441, -5.622872871577872189 ) ) ;
#2942=EDGE_LOOP ( 'NONE', ( #20773, #11386, #17741, #16971 ) ) ;
#2945=CARTESIAN_POINT ( 'NONE',  ( -5.444914386472299306, 34.55078125108393294, 13.14518615778179722 ) ) ;
#2946=CARTESIAN_POINT ( 'NONE',  ( -9.598844408820458085, 33.06250000216787299, -9.598844408820458085 ) ) ;
#2965=CARTESIAN_POINT ( 'NONE',  ( -13.14518615778179900, 36.53515625108392584, -5.444914386472297529 ) ) ;
#2998=CARTESIAN_POINT ( 'NONE',  ( -5.444914386472297529, 34.05468750108393294, -13.14518615778179722 ) ) ;
#3008=CARTESIAN_POINT ( 'NONE',  ( 0.000000000000000000, 30.99999999999999645, 0.000000000000000000 ) ) ;
#3019=CARTESIAN_POINT ( 'NONE',  ( 13.57481594606304753, 39.95820312716787726, -5.622872871577873966 ) ) ;
#3041=CARTESIAN_POINT ( 'NONE',  ( 2.414731522848535132E-15, 36.98164062608393721, 13.14518615778179544 ) ) ;
#3049=CARTESIAN_POINT ( 'NONE',  ( 9.295050272127047819, 34.69960937608393436, 9.295050272127046043 ) ) ;
#3057=CARTESIAN_POINT ( 'NONE',  ( -9.598844408820454532, 33.16171874999999858, 9.598844408820459861 ) ) ;
#3058=CARTESIAN_POINT ( 'NONE',  ( -13.14518615778179544, 32.61601562608393579, 0.000000000000000000 ) ) ;
#3073=CARTESIAN_POINT ( 'NONE',  ( -8.312177448680279460E-16, 32.16953125216787157, -13.57481594606304576 ) ) ;
#3077=PRESENTATION_STYLE_ASSIGNMENT (( #806 ) ) ;
#3093=ORIENTED_EDGE ( 'NONE', *, *, #13327, .F. ) ;
#3095=CARTESIAN_POINT ( 'NONE',  ( -5.444914386472297529, 33.45937500108394147, -13.14518615778179900 ) ) ;
#3096=CARTESIAN_POINT ( 'NONE',  ( -5.622872871577873077, 34.60039062716786873, -13.57481594606304753 ) ) ;
#3105=CARTESIAN_POINT ( 'NONE',  ( 2.493653234604083739E-15, 38.91640625216786731, 13.57481594606304576 ) ) ;
#3107=CARTESIAN_POINT ( 'NONE',  ( -8.312177448680279460E-16, 31.37578125216787583, -13.57481594606304576 ) ) ;
#3115=CARTESIAN_POINT ( 'NONE',  ( 1.662435489736055892E-15, 40.99999999999999289, 13.57481594606304576 ) ) ;
#3117=CARTESIAN_POINT ( 'NONE',  ( -5.444914386472299306, 33.55859375108393294, 13.14518615778179722 ) ) ;
#3121=CARTESIAN_POINT ( 'NONE',  ( -8.312177448680279460E-16, 37.72578125216787726, -13.57481594606304576 ) ) ;
#3149=CARTESIAN_POINT ( 'NONE',  ( -8.049105076161786076E-16, 32.41757812608393863, -13.14518615778179544 ) ) ;
#3154=CARTESIAN_POINT ( 'NONE',  ( 5.622872871578008080, 36.08867187716787583, -13.57481594606290898 ) ) ;
#3185=CARTESIAN_POINT ( 'NONE',  ( -5.444914386472299306, 35.34453125108393579, 13.14518615778179722 ) ) ;
#3190=CARTESIAN_POINT ( 'NONE',  ( 13.14518615778179722, 35.54296875108394715, 5.444914386472293977 ) ) ;
#3196=CARTESIAN_POINT ( 'NONE',  ( 5.622872871577878406, 34.10429687499999574, 13.57481594606304576 ) ) ;
#3197=CARTESIAN_POINT ( 'NONE',  ( -5.444914386472297529, 34.84843750108393579, -13.14518615778179900 ) ) ;
#3209=ADVANCED_FACE ( 'NONE', ( #19413 ), #19987, .F. ) ;
#3211=CARTESIAN_POINT ( 'NONE',  ( -13.57481594606304576, 34.74921875216787726, 0.000000000000000000 ) ) ;
#3212=CARTESIAN_POINT ( 'NONE',  ( 7.095735352922348582, 31.91687086491026193, -11.40432286404674933 ) ) ;
#3226=CARTESIAN_POINT ( 'NONE',  ( 5.622872871577825116, 35.29492187716787299, -13.57481594606309372 ) ) ;
#3230=ORIENTED_EDGE ( 'NONE', *, *, #9027, .T. ) ;
#3232=CARTESIAN_POINT ( 'NONE',  ( -13.14518615778179900, 35.14609375108393152, -5.444914386472297529 ) ) ;
#3233=CARTESIAN_POINT ( 'NONE',  ( 5.622872871577878406, 32.61601562716786873, 13.57481594606304576 ) ) ;
#3234=( BOUNDED_CURVE ( )  B_SPLINE_CURVE ( 2, ( #3121, #18074, #22220, #20512, #994, #18365, #24919, #1135, #5403 ),
 .UNSPECIFIED., .F., .F. ) 
 B_SPLINE_CURVE_WITH_KNOTS ( ( 3, 2, 2, 2, 3 ),
 ( 0.2708333333333330928, 0.2812499999999998890, 0.2916666666666666852, 0.3020833333333334259, 0.3125000000000002220 ),
 .UNSPECIFIED. ) 
 CURVE ( )  GEOMETRIC_REPRESENTATION_ITEM ( )  RATIONAL_B_SPLINE_CURVE ( ( 1.000000000000001554, 0.9238795325112850731, 1.000000000000000000, 0.9238795325112867385, 1.000000000000000000, 0.9238795325112867385, 1.000000000000000000, 0.9238795325112850731, 1.000000000000001554 ) ) 
 REPRESENTATION_ITEM ( '' )  );
#3238=VECTOR ( 'NONE', #7754, 1000.000000000000000 ) ;
#3251=EDGE_CURVE ( 'NONE', #23528, #10223, #4739, .T. ) ;
#3259=CARTESIAN_POINT ( 'NONE',  ( -13.14518615778179544, 31.82226562608393650, 0.000000000000000000 ) ) ;
#3262=CARTESIAN_POINT ( 'NONE',  ( 2.493653234604083739E-15, 38.12265625216787157, 13.57481594606304576 ) ) ;
#3306=LINE ( 'NONE', #7423, #15196 ) ;
#3323=CARTESIAN_POINT ( 'NONE',  ( -9.295050272127044266, 32.11992187608393579, 9.295050272127047819 ) ) ;
#3330=CARTESIAN_POINT ( 'NONE',  ( -13.14518615778179189, 35.24531250108393721, 5.444914386472304635 ) ) ;
#3341=CARTESIAN_POINT ( 'NONE',  ( 9.598844408820459861, 32.66562500216787157, 9.598844408820456309 ) ) ;
#3350=CARTESIAN_POINT ( 'NONE',  ( 13.57481594606304931, 31.92148437716787157, 5.622872871577868636 ) ) ;
#3356=DIRECTION ( 'NONE',  ( 0.000000000000000000, 1.000000000000000000, 0.000000000000000000 ) ) ;
#3364=VERTEX_POINT ( 'NONE', #4315 ) ;
#3366=CARTESIAN_POINT ( 'NONE',  ( -13.14518615778179544, 35.19570312608393436, 0.000000000000000000 ) ) ;
#3367=CARTESIAN_POINT ( 'NONE',  ( -8.312177448680279460E-16, 34.55078125216787299, -13.57481594606304576 ) ) ;
#3388=CARTESIAN_POINT ( 'NONE',  ( -13.57481594606304398, 33.11210937499999574, 5.622872871577880183 ) ) ;
#3390=CARTESIAN_POINT ( 'NONE',  ( 9.295050272127047819, 32.91367187608393152, 9.295050272127046043 ) ) ;
#3417=ADVANCED_FACE ( 'NONE', ( #5165 ), #22698, .F. ) ;
#3425=CARTESIAN_POINT ( 'NONE',  ( 6.944423797152706079, 31.55306878032414986, -11.16113333171310451 ) ) ;
#3456=CARTESIAN_POINT ( 'NONE',  ( 13.14518615778179722, 40.10703125108393152, 5.444914386472293977 ) ) ;
#3463=CARTESIAN_POINT ( 'NONE',  ( -5.444914386472299306, 33.75703125108393721, 13.14518615778179722 ) ) ;
#3470=CARTESIAN_POINT ( 'NONE',  ( 13.14518615778179544, 34.00507812608393721, -1.609821015232357215E-15 ) ) ;
#3492=DIRECTION ( 'NONE',  ( -0.5282856486898074300, 0.000000000000000000, 0.8490667072665075699 ) ) ;
#3507=CARTESIAN_POINT ( 'NONE',  ( -13.14518615778179544, 40.75195312608393294, 0.000000000000000000 ) ) ;
#3511=PRODUCT_DEFINITION_CONTEXT ( 'detailed design', #1690, 'design' ) ;
#3512=CARTESIAN_POINT ( 'NONE',  ( 9.598844408820456309, 38.32109374999999574, -9.598844408820458085 ) ) ;
#3513=CARTESIAN_POINT ( 'NONE',  ( 5.444914386472302859, 40.00781250108393294, 13.14518615778179189 ) ) ;
#3519=ORIENTED_EDGE ( 'NONE', *, *, #18368, .F. ) ;
#3555=CARTESIAN_POINT ( 'NONE',  ( -13.57481594606304753, 39.46210937716787726, -5.622872871577873077 ) ) ;
#3566=CARTESIAN_POINT ( 'NONE',  ( -8.312177448680279460E-16, 31.37578125216787583, -13.57481594606304576 ) ) ;
#3595=EDGE_CURVE ( 'NONE', #10432, #10042, #3306, .T. ) ;
#3600=CARTESIAN_POINT ( 'NONE',  ( 9.295050272127046043, 39.46210937608393010, -9.295050272127046043 ) ) ;
#3609=CARTESIAN_POINT ( 'NONE',  ( 5.444914386472297529, 34.15390625108393863, -13.14518615778179900 ) ) ;
#3616=CARTESIAN_POINT ( 'NONE',  ( 5.444914386472302859, 33.06250000108393294, 13.14518615778179189 ) ) ;
#3622=CARTESIAN_POINT ( 'NONE',  ( 3.755638265659908104, 31.58960998161716560, -13.14518615778179900 ) ) ;
#3641=CARTESIAN_POINT ( 'NONE',  ( 2.493653234604083739E-15, 33.26093749999999716, 13.57481594606304576 ) ) ;
#3644=CARTESIAN_POINT ( 'NONE',  ( -8.049105076161786076E-16, 40.55351562608393579, -13.14518615778179544 ) ) ;
#3654=CARTESIAN_POINT ( 'NONE',  ( -13.57481594606304576, 39.46210937499999005, 5.622872871577880183 ) ) ;
#3655=CARTESIAN_POINT ( 'NONE',  ( 9.295050272127046043, 39.46210937608393010, -9.295050272127046043 ) ) ;
#3669=VERTEX_POINT ( 'NONE', #22979 ) ;
#3694=CARTESIAN_POINT ( 'NONE',  ( -13.14518615778179544, 39.95820312608393010, 0.000000000000000000 ) ) ;
#3722=CARTESIAN_POINT ( 'NONE',  ( 13.57481594606304931, 39.75976562499999289, 5.622872871577868636 ) ) ;
#3725=ORIENTED_EDGE ( 'NONE', *, *, #2373, .T. ) ;
#3737=CARTESIAN_POINT ( 'NONE',  ( 9.295050272127047819, 40.05742187608392868, 9.295050272127046043 ) ) ;
#3747=CARTESIAN_POINT ( 'NONE',  ( -5.444914386472297529, 34.25312500108393010, -13.14518615778179900 ) ) ;
#3753=ORIENTED_EDGE ( 'NONE', *, *, #11729, .F. ) ;
#3754=CARTESIAN_POINT ( 'NONE',  ( -13.14518615778179544, 32.02070312608393010, 0.000000000000000000 ) ) ;
#3756=EDGE_CURVE ( 'NONE', #13728, #10337, #8134, .T. ) ;
#3789=CARTESIAN_POINT ( 'NONE',  ( -5.622872871577873077, 40.05742187499999574, -13.57481594606304753 ) ) ;
#3790=CARTESIAN_POINT ( 'NONE',  ( 13.57481594606304576, 31.97109375216787441, -1.662435489736055892E-15 ) ) ;
#3809=CARTESIAN_POINT ( 'NONE',  ( -13.57481594606304398, 32.41757812716787868, 5.622872871577880183 ) ) ;
#3826=CARTESIAN_POINT ( 'NONE',  ( 5.444914386472297529, 39.71015625108393010, -13.14518615778179900 ) ) ;
#3827=CARTESIAN_POINT ( 'NONE',  ( -8.312177448680279460E-16, 40.10703125216787157, -13.57481594606304576 ) ) ;
#3844=FACE_OUTER_BOUND ( 'NONE', #19807, .T. ) ;
#3864=CARTESIAN_POINT ( 'NONE',  ( -9.598844408820458085, 33.06250000216787299, -9.598844408820458085 ) ) ;
#3870=CARTESIAN_POINT ( 'NONE',  ( 5.444914386472302859, 40.00781250108393294, 13.14518615778179189 ) ) ;
#3882=CARTESIAN_POINT ( 'NONE',  ( -13.14518615778179544, 32.81445312608393294, 0.000000000000000000 ) ) ;
#3889=CARTESIAN_POINT ( 'NONE',  ( 13.14518615778179722, 32.36796875108393579, 5.444914386472293977 ) ) ;
#3895=CARTESIAN_POINT ( 'NONE',  ( -9.598844408820454532, 32.36796874999999574, 9.598844408820459861 ) ) ;
#3899=CARTESIAN_POINT ( 'NONE',  ( 2.493653234604083739E-15, 34.84843749999999574, 13.57481594606304576 ) ) ;
#3901=ORIENTED_EDGE ( 'NONE', *, *, #11311, .F. ) ;
#3913=EDGE_CURVE ( 'NONE', #10042, #17637, #8373, .T. ) ;
#3914=VERTEX_POINT ( 'NONE', #20803 ) ;
#3915=CARTESIAN_POINT ( 'NONE',  ( -13.14518615778179189, 33.45937500108392726, 5.444914386472304635 ) ) ;
#3930=CARTESIAN_POINT ( 'NONE',  ( 13.57481594606304753, 39.85898437499999858, -5.622872871577873077 ) ) ;
#3931=CARTESIAN_POINT ( 'NONE',  ( -5.444914386472297529, 38.81718750108393579, -13.14518615778179900 ) ) ;
#3949=EDGE_CURVE ( 'NONE', #21855, #19872, #18453, .T. ) ;
#3980=CLOSED_SHELL ( 'NONE', ( #3417, #18569, #824, #23023, #19804, #19694, #21880, #22070, #12567, #8474, #205, #21637, #26572, #19130, #7546, #12067, #18198, #3209, #6160, #23117, #22791, #9244, #12595, #12804, #18563, #25354, #460, #26694, #24822, #16692, #11939, #21191, #12947, #11029 ) ) ;
#3988=CARTESIAN_POINT ( 'NONE',  ( -8.049105076161786076E-16, 40.35507812608393152, -13.14518615778179544 ) ) ;
#4013=CARTESIAN_POINT ( 'NONE',  ( 13.14518615778179722, 38.51953125108393294, 5.444914386472293977 ) ) ;
#4049=VECTOR ( 'NONE', #16493, 1000.000000000000000 ) ;
#4057=CARTESIAN_POINT ( 'NONE',  ( -13.14518615778179544, 38.37070312608393152, 0.000000000000000000 ) ) ;
#4070=CARTESIAN_POINT ( 'NONE',  ( 2.493653234604083739E-15, 38.81718749999999574, 13.57481594606304576 ) ) ;
#4071=CARTESIAN_POINT ( 'NONE',  ( 13.14518615778179900, 40.20625000108393010, -5.444914386472297529 ) ) ;
#4080=CARTESIAN_POINT ( 'NONE',  ( -13.57481594606304753, 38.66835937716787441, -5.622872871577872189 ) ) ;
#4081=CYLINDRICAL_SURFACE ( 'NONE', #8078, 13.57481594606304576 ) ;
#4086=LINE ( 'NONE', #5946, #14603 ) ;
#4101=CARTESIAN_POINT ( 'NONE',  ( -5.622872871577767384, 40.85117187499999147, -13.57481594606315412 ) ) ;
#4106=CARTESIAN_POINT ( 'NONE',  ( 9.295050272127047819, 39.46210937608393721, 9.295050272127046043 ) ) ;
#4107=CARTESIAN_POINT ( 'NONE',  ( -13.57481594606304576, 39.51171875216787299, 0.000000000000000000 ) ) ;
#4117=CARTESIAN_POINT ( 'NONE',  ( -8.312177448680279460E-16, 38.42031249999999432, -13.57481594606304576 ) ) ;
#4125=CARTESIAN_POINT ( 'NONE',  ( 13.14518615778179900, 38.51953125108393294, 5.444914386472293977 ) ) ;
#4127=CARTESIAN_POINT ( 'NONE',  ( 13.57481594606304576, 35.84062499999999574, -1.662435489736055892E-15 ) ) ;
#4154=CARTESIAN_POINT ( 'NONE',  ( 2.414731522848535132E-15, 37.57695312608392868, 13.14518615778179544 ) ) ;
#4164=CARTESIAN_POINT ( 'NONE',  ( 2.493653234604083739E-15, 34.84843749999999574, 13.57481594606304576 ) ) ;
#4168=CYLINDRICAL_SURFACE ( 'NONE', #26722, 13.57481594606304576 ) ;
#4183=CARTESIAN_POINT ( 'NONE',  ( -8.312177448680279460E-16, 33.75703125216787726, -13.57481594606304576 ) ) ;
#4189=ORIENTED_EDGE ( 'NONE', *, *, #3756, .F. ) ;
#4192=ORIENTED_EDGE ( 'NONE', *, *, #16531, .F. ) ;
#4194=CARTESIAN_POINT ( 'NONE',  ( 5.444914386472297529, 38.12265625108393152, -13.14518615778179900 ) ) ;
#4205=CARTESIAN_POINT ( 'NONE',  ( -9.598844408820454532, 37.13046874999999147, 9.598844408820459861 ) ) ;
#4206=CARTESIAN_POINT ( 'NONE',  ( 2.414731522848535132E-15, 35.98945312608393010, 13.14518615778179544 ) ) ;
#4216=CARTESIAN_POINT ( 'NONE',  ( -5.622872871578011633, 38.86679687716787868, 13.57481594606290720 ) ) ;
#4241=DIRECTION ( 'NONE',  ( 0.000000000000000000, 0.000000000000000000, -1.000000000000000000 ) ) ;
#4242=CARTESIAN_POINT ( 'NONE',  ( 9.295050272127046043, 36.48554687608393721, -9.295050272127046043 ) ) ;
#4243=CARTESIAN_POINT ( 'NONE',  ( -5.622872871577873077, 36.48554687716787015, 13.57481594606304753 ) ) ;
#4250=ORIENTED_EDGE ( 'NONE', *, *, #22553, .F. ) ;
#4255=DIRECTION ( 'NONE',  ( -0.000000000000000000, -1.000000000000000000, -0.000000000000000000 ) ) ;
#4289=CARTESIAN_POINT ( 'NONE',  ( 13.14518615778179722, 35.44375000108393436, -5.444914386472297529 ) ) ;
#4304=EDGE_CURVE ( 'NONE', #947, #15078, #18125, .T. ) ;
#4315=CARTESIAN_POINT ( 'NONE',  ( -8.312177448680279460E-16, 35.34453125216787583, -13.57481594606304576 ) ) ;
#4332=CARTESIAN_POINT ( 'NONE',  ( 9.295050272127047819, 38.66835937608393436, 9.295050272127046043 ) ) ;
#4338=CARTESIAN_POINT ( 'NONE',  ( -5.444914386472299306, 39.31328125108392868, 13.14518615778179722 ) ) ;
#4345=CARTESIAN_POINT ( 'NONE',  ( -13.57481594606304576, 37.08085937499999574, 5.622872871577880183 ) ) ;
#4346=CARTESIAN_POINT ( 'NONE',  ( -5.444914386472299306, 37.52734375108393294, 13.14518615778179722 ) ) ;
#4363=CARTESIAN_POINT ( 'NONE',  ( -8.312177448680279460E-16, 36.83281249999999574, -13.57481594606304576 ) ) ;
#4377=EDGE_LOOP ( 'NONE', ( #1231, #15868, #14798, #15280 ) ) ;
#4378=CARTESIAN_POINT ( 'NONE',  ( -13.57481594606304398, 39.46210937499999005, 5.622872871577880183 ) ) ;
#4384=CARTESIAN_POINT ( 'NONE',  ( 5.444914386472297529, 36.53515625108393294, -13.14518615778179900 ) ) ;
#4385=CARTESIAN_POINT ( 'NONE',  ( 13.57481594606304753, 38.37070312716786447, -5.622872871577873077 ) ) ;
#4403=AXIS2_PLACEMENT_3D ( 'NONE', #14813, #21261, #6556 ) ;
#4405=CARTESIAN_POINT ( 'NONE',  ( 5.444914386472297529, 38.71796875108393721, -13.14518615778179900 ) ) ;
#4408=CARTESIAN_POINT ( 'NONE',  ( 13.57481594606304753, 39.06523437499999574, -5.622872871577873966 ) ) ;
#4418=VECTOR ( 'NONE', #17117, 1000.000000000000000 ) ;
#4431=VERTEX_POINT ( 'NONE', #975 ) ;
#4435=CARTESIAN_POINT ( 'NONE',  ( -13.14518615778179722, 34.94765625108394147, -5.444914386472297529 ) ) ;
#4462=ORIENTED_EDGE ( 'NONE', *, *, #14513, .F. ) ;
#4464=CARTESIAN_POINT ( 'NONE',  ( 13.57481594606304931, 33.50898437716787015, 5.622872871577868636 ) ) ;
#4475=ORIENTED_EDGE ( 'NONE', *, *, #21691, .T. ) ;
#4476=CARTESIAN_POINT ( 'NONE',  ( -5.444914386472299306, 37.72578125108395142, 13.14518615778179722 ) ) ;
#4482=CARTESIAN_POINT ( 'NONE',  ( -9.295050272127046043, 37.47773437608393010, -9.295050272127046043 ) ) ;
#4484=LINE ( 'NONE', #22011, #2089 ) ;
#4489=CARTESIAN_POINT ( 'NONE',  ( -9.598844408820454532, 36.33671874999999574, 9.598844408820459861 ) ) ;
#4490=CARTESIAN_POINT ( 'NONE',  ( 9.295050272127047819, 36.88242187608393152, 9.295050272127046043 ) ) ;
#4502=DIRECTION ( 'NONE',  ( 0.000000000000000000, 1.000000000000000000, 0.000000000000000000 ) ) ;
#4513=CARTESIAN_POINT ( 'NONE',  ( 5.622872871577733633, 32.81445312500000000, -13.57481594606318254 ) ) ;
#4521=ORIENTED_EDGE ( 'NONE', *, *, #20656, .T. ) ;
#4522=DIRECTION ( 'NONE',  ( -0.000000000000000000, -1.000000000000000000, -0.000000000000000000 ) ) ;
#4523=CARTESIAN_POINT ( 'NONE',  ( -9.295050272127044266, 36.08867187608393579, 9.295050272127047819 ) ) ;
#4524=CARTESIAN_POINT ( 'NONE',  ( -8.312177448680279460E-16, 36.93203125216787441, -13.57481594606304576 ) ) ;
#4533=CARTESIAN_POINT ( 'NONE',  ( -5.622872871577873966, 34.10429687716786873, 13.57481594606304753 ) ) ;
#4543=CARTESIAN_POINT ( 'NONE',  ( 13.14518615778179544, 35.39414062608393152, -1.609821015232357215E-15 ) ) ;
#4555=ORIENTED_EDGE ( 'NONE', *, *, #28182, .F. ) ;
#4571=CARTESIAN_POINT ( 'NONE',  ( 5.444914386472297529, 34.74921875108393721, -13.14518615778179722 ) ) ;
#4572=CARTESIAN_POINT ( 'NONE',  ( 13.57481594606304576, 36.73359375216787015, -1.662435489736055892E-15 ) ) ;
#4614=CARTESIAN_POINT ( 'NONE',  ( -13.14518615778179900, 40.70234375108393721, -5.444914386472297529 ) ) ;
#4622=CARTESIAN_POINT ( 'NONE',  ( 13.14518615778179544, 37.97382812608393721, -1.609821015232357215E-15 ) ) ;
#4623=CARTESIAN_POINT ( 'NONE',  ( -9.598844408820458085, 39.41250000216787441, -9.598844408820458085 ) ) ;
#4629=CARTESIAN_POINT ( 'NONE',  ( -13.57481594606304753, 37.77539062499999289, -5.622872871577873077 ) ) ;
#4630=CARTESIAN_POINT ( 'NONE',  ( 9.295050272127046043, 37.87460937608393152, -9.295050272127046043 ) ) ;
#4642=DIRECTION ( 'NONE',  ( -0.000000000000000000, -1.000000000000000000, -0.000000000000000000 ) ) ;
#4660=CARTESIAN_POINT ( 'NONE',  ( -9.598844408820458085, 39.31328124999999574, -9.598844408820458085 ) ) ;
#4668=CARTESIAN_POINT ( 'NONE',  ( 2.414731522848535132E-15, 36.18789062608393436, 13.14518615778179544 ) ) ;
#4669=CARTESIAN_POINT ( 'NONE',  ( 13.57481594606304931, 35.89023437716787868, 5.622872871577869525 ) ) ;
#4673=ORIENTED_EDGE ( 'NONE', *, *, #24988, .F. ) ;
#4683=EDGE_LOOP ( 'NONE', ( #3093, #27484, #23816, #13395, #7616, #6409, #19558, #3230, #10808, #14475, #6143, #20661, #26578, #15872, #10954, #10552, #12434, #22524, #24367, #1816, #14565, #11686, #25757, #16477, #5639, #937, #20308 ) ) ;
#4689=CARTESIAN_POINT ( 'NONE',  ( 9.295050272127047819, 35.29492187608393294, 9.295050272127046043 ) ) ;
#4706=CIRCLE ( 'NONE', #1519, 15.57481594606304576 ) ;
#4715=UNCERTAINTY_MEASURE_WITH_UNIT (LENGTH_MEASURE( 1.000000000000000082E-05 ), #4934, 'distance_accuracy_value', 'NONE');
#4718=CARTESIAN_POINT ( 'NONE',  ( -13.14518615778179544, 36.58476562608393579, 0.000000000000000000 ) ) ;
#4739=LINE ( 'NONE', #2460, #20699 ) ;
#4742=CARTESIAN_POINT ( 'NONE',  ( 2.493653234604083739E-15, 32.46718749999999432, 13.57481594606304576 ) ) ;
#4759=CARTESIAN_POINT ( 'NONE',  ( 5.444914386472302859, 35.44375000108393436, 13.14518615778179189 ) ) ;
#4764=CARTESIAN_POINT ( 'NONE',  ( -13.14518615778179189, 36.83281250108393579, 5.444914386472304635 ) ) ;
#4771=CARTESIAN_POINT ( 'NONE',  ( 9.598844408820456309, 35.14609374999999858, -9.598844408820458085 ) ) ;
#4772=CARTESIAN_POINT ( 'NONE',  ( -9.295050272127044266, 38.27148437608393294, 9.295050272127047819 ) ) ;
#4784=CARTESIAN_POINT ( 'NONE',  ( 1.662435489736055892E-15, 40.99999999999999289, 13.57481594606304576 ) ) ;
#4787=CARTESIAN_POINT ( 'NONE',  ( -8.312177448680279460E-16, 36.83281249999999574, -13.57481594606304576 ) ) ;
#4798=CARTESIAN_POINT ( 'NONE',  ( 9.598844408820459861, 32.56640625000000000, 9.598844408820456309 ) ) ;
#4810=CARTESIAN_POINT ( 'NONE',  ( 13.14518615778179544, 35.59257812608393579, -1.609821015232357215E-15 ) ) ;
#4811=CARTESIAN_POINT ( 'NONE',  ( -5.622872871577873077, 38.86679687716788578, 13.57481594606304753 ) ) ;
#4836=CARTESIAN_POINT ( 'NONE',  ( -13.14518615778179544, 35.79101562608393294, 0.000000000000000000 ) ) ;
#4840=DIRECTION ( 'NONE',  ( 1.000000000000000000, 0.000000000000000000, 0.000000000000000000 ) ) ;
#4846=ORIENTED_EDGE ( 'NONE', *, *, #11204, .T. ) ;
#4863=CARTESIAN_POINT ( 'NONE',  ( -9.295050272127044266, 33.50898437608393010, 9.295050272127047819 ) ) ;
#4905=CARTESIAN_POINT ( 'NONE',  ( 5.444914386472297529, 36.53515625108393294, -13.14518615778179900 ) ) ;
#4911=CARTESIAN_POINT ( 'NONE',  ( -5.444914386472299306, 36.93203125108394147, 13.14518615778179722 ) ) ;
#4914=CARTESIAN_POINT ( 'NONE',  ( -13.57481594606304576, 36.23749999999999005, 0.000000000000000000 ) ) ;
#4918=CARTESIAN_POINT ( 'NONE',  ( 9.598844408820459861, 34.94765624999999432, 9.598844408820456309 ) ) ;
#4919=CARTESIAN_POINT ( 'NONE',  ( 13.14518615778179900, 35.34453125108392868, 5.444914386472293977 ) ) ;
#4932=CARTESIAN_POINT ( 'NONE',  ( 7.020079488845731852, 31.83418857360491216, -11.28272815150820563 ) ) ;
#4934=( LENGTH_UNIT ( ) NAMED_UNIT ( * ) SI_UNIT ( .MILLI., .METRE. ) );
#4936=ORIENTED_EDGE ( 'NONE', *, *, #6390, .T. ) ;
#4955=CARTESIAN_POINT ( 'NONE',  ( 5.444914386472297529, 34.94765625108394147, -13.14518615778179900 ) ) ;
#4956=CARTESIAN_POINT ( 'NONE',  ( 13.57481594606304931, 34.30273437716787299, 5.622872871577869525 ) ) ;
#4976=CARTESIAN_POINT ( 'NONE',  ( -9.295050272127044266, 37.47773437608393010, 9.295050272127047819 ) ) ;
#4984=ORIENTED_EDGE ( 'NONE', *, *, #26043, .T. ) ;
#5007=CARTESIAN_POINT ( 'NONE',  ( 9.295050272127046043, 33.11210937608393579, -9.295050272127046043 ) ) ;
#5045=CARTESIAN_POINT ( 'NONE',  ( -13.14518615778179189, 36.03906250108394005, 5.444914386472304635 ) ) ;
#5050=CARTESIAN_POINT ( 'NONE',  ( -9.295050272127044266, 34.50117187608393721, 9.295050272127047819 ) ) ;
#5058=CARTESIAN_POINT ( 'NONE',  ( 13.57481594606304931, 34.20351562499999432, 5.622872871577869525 ) ) ;
#5059=CARTESIAN_POINT ( 'NONE',  ( -5.444914386472299306, 33.55859375108393294, 13.14518615778179722 ) ) ;
#5073=CARTESIAN_POINT ( 'NONE',  ( 2.493653234604083739E-15, 34.94765625216787441, 13.57481594606304576 ) ) ;
#5091=ORIENTED_EDGE ( 'NONE', *, *, #18034, .T. ) ;
#5093=CARTESIAN_POINT ( 'NONE',  ( -8.049105076161786076E-16, 34.99726562608393721, -13.14518615778179544 ) ) ;
#5094=CARTESIAN_POINT ( 'NONE',  ( 2.493653234604083739E-15, 34.94765625216787441, 13.57481594606304576 ) ) ;
#5113=CARTESIAN_POINT ( 'NONE',  ( 2.414731522848535132E-15, 35.98945312608393010, 13.14518615778179544 ) ) ;
#5120=CARTESIAN_POINT ( 'NONE',  ( -9.598844408820458085, 35.44375000216787441, -9.598844408820458085 ) ) ;
#5138=ORIENTED_EDGE ( 'NONE', *, *, #22744, .F. ) ;
#5142=CARTESIAN_POINT ( 'NONE',  ( -13.14518615778179189, 33.45937500108393436, 5.444914386472304635 ) ) ;
#5164=CARTESIAN_POINT ( 'NONE',  ( -8.312177448680279460E-16, 40.10703125216787157, -13.57481594606304576 ) ) ;
#5165=FACE_OUTER_BOUND ( 'NONE', #25670, .T. ) ;
#5186=CARTESIAN_POINT ( 'NONE',  ( -5.444914386472297529, 35.84062500108394289, -13.14518615778179900 ) ) ;
#5191=CARTESIAN_POINT ( 'NONE',  ( -9.295050272127046043, 35.09648437608393579, -9.295050272127046043 ) ) ;
#5194=CARTESIAN_POINT ( 'NONE',  ( -13.57481594606304753, 36.18789062499999432, -5.622872871577872189 ) ) ;
#5198=CARTESIAN_POINT ( 'NONE',  ( 9.598844408820459861, 33.36015624999999574, 9.598844408820456309 ) ) ;
#5199=CARTESIAN_POINT ( 'NONE',  ( -5.444914386472299306, 32.76484375108393010, 13.14518615778179722 ) ) ;
#5213=CARTESIAN_POINT ( 'NONE',  ( 5.622872871577832221, 36.48554687499999716, 13.57481594606309194 ) ) ;
#5233=CARTESIAN_POINT ( 'NONE',  ( 13.14518615778179900, 34.05468750108394005, -5.444914386472297529 ) ) ;
#5234=CARTESIAN_POINT ( 'NONE',  ( 9.598844408820456309, 33.65781250216787157, -9.598844408820458085 ) ) ;
#5254=CARTESIAN_POINT ( 'NONE',  ( 13.57481594606304931, 40.55351562499999574, 5.622872871577868636 ) ) ;
#5256=CARTESIAN_POINT ( 'NONE',  ( -5.444914386472297529, 34.05468750108393294, -13.14518615778179900 ) ) ;
#5262=CARTESIAN_POINT ( 'NONE',  ( 0.000000000000000000, 40.99999999999999289, -13.57481594606304576 ) ) ;
#5263=CARTESIAN_POINT ( 'NONE',  ( -13.36000105192242060, 40.42949218912590936, 0.000000000000000000 ) ) ;
#5285=CARTESIAN_POINT ( 'NONE',  ( 5.444914386472297529, 33.95546875108394147, -13.14518615778179722 ) ) ;
#5306=CARTESIAN_POINT ( 'NONE',  ( 13.57481594606304931, 39.85898437716787157, 5.622872871577868636 ) ) ;
#5311=VERTEX_POINT ( 'NONE', #18832 ) ;
#5317=VECTOR ( 'NONE', #20065, 1000.000000000000000 ) ;
#5327=CARTESIAN_POINT ( 'NONE',  ( -13.14518615778179544, 34.40195312608393152, 0.000000000000000000 ) ) ;
#5334=CARTESIAN_POINT ( 'NONE',  ( -13.14518615778179189, 36.03906250108393294, 5.444914386472304635 ) ) ;
#5340=CARTESIAN_POINT ( 'NONE',  ( -9.598844408820454532, 32.36796874999999574, 9.598844408820459861 ) ) ;
#5341=CARTESIAN_POINT ( 'NONE',  ( 13.14518615778179544, 35.39414062608393152, -1.609821015232357215E-15 ) ) ;
#5344=CARTESIAN_POINT ( 'NONE',  ( 7.095734625815413921, 31.38770419771516629, -11.40432331644931629 ) ) ;
#5377=CARTESIAN_POINT ( 'NONE',  ( -8.049105076161786076E-16, 34.20351562608394147, -13.14518615778179544 ) ) ;
#5378=CARTESIAN_POINT ( 'NONE',  ( -13.57481594606304753, 35.49335937716787015, -5.622872871577873077 ) ) ;
#5400=CARTESIAN_POINT ( 'NONE',  ( -13.14518615778179189, 31.87187500108393223, 5.444914386472304635 ) ) ;
#5403=CARTESIAN_POINT ( 'NONE',  ( 2.493653234604083739E-15, 37.32890625216786873, 13.57481594606304576 ) ) ;
#5420=CIRCLE ( 'NONE', #21330, 13.57481594606304576 ) ;
#5429=CARTESIAN_POINT ( 'NONE',  ( -13.14518615778179544, 31.82226562608393650, 0.000000000000000000 ) ) ;
#5443=CARTESIAN_POINT ( 'NONE',  ( 13.57481594606304753, 39.85898437499999858, -5.622872871577873966 ) ) ;
#5456=( BOUNDED_CURVE ( )  B_SPLINE_CURVE ( 2, ( #7067, #18046, #26474, #20339, #19910 ),
 .UNSPECIFIED., .F., .F. ) 
 B_SPLINE_CURVE_WITH_KNOTS ( ( 3, 2, 3 ),
 ( 0.000000000000000000, 0.01041666666666679446, 0.02083333333333358892 ),
 .UNSPECIFIED. ) 
 CURVE ( )  GEOMETRIC_REPRESENTATION_ITEM ( )  RATIONAL_B_SPLINE_CURVE ( ( 1.000000000000000000, 0.9238795325112867385, 1.000000000000000000, 0.9238795325112848511, 1.000000000000001776 ) ) 
 REPRESENTATION_ITEM ( '' )  );
#5466=CARTESIAN_POINT ( 'NONE',  ( 13.57481594606304576, 38.32109375216786873, -1.662435489736055892E-15 ) ) ;
#5474=CARTESIAN_POINT ( 'NONE',  ( 9.295050272127047819, 35.49335937608393721, 9.295050272127046043 ) ) ;
#5480=CARTESIAN_POINT ( 'NONE',  ( 9.598844408820459861, 32.56640625000000000, 9.598844408820456309 ) ) ;
#5481=CARTESIAN_POINT ( 'NONE',  ( 13.14518615778179544, 33.80664062608393294, -1.609821015232357215E-15 ) ) ;
#5483=DIRECTION ( 'NONE',  ( -0.000000000000000000, -1.000000000000000000, -0.000000000000000000 ) ) ;
#5518=CARTESIAN_POINT ( 'NONE',  ( 2.414731522848535132E-15, 34.60039062608393579, 13.14518615778179544 ) ) ;
#5519=CARTESIAN_POINT ( 'NONE',  ( 5.622872871577871301, 35.29492187716788720, -13.57481594606304753 ) ) ;
#5530=VECTOR ( 'NONE', #5854, 1000.000000000000000 ) ;
#5543=CARTESIAN_POINT ( 'NONE',  ( 2.493653234604083739E-15, 33.26093749999999716, 13.57481594606304576 ) ) ;
#5545=CARTESIAN_POINT ( 'NONE',  ( -5.444914386472297529, 32.46718750108393436, -13.14518615778179900 ) ) ;
#5570=VERTEX_POINT ( 'NONE', #12835 ) ;
#5592=DIRECTION ( 'NONE',  ( -0.8660254037844407060, 0.4999999999999963363, 0.000000000000000000 ) ) ;
#5609=CARTESIAN_POINT ( 'NONE',  ( 9.295050272127046043, 32.51679687608393721, -9.295050272127046043 ) ) ;
#5616=CARTESIAN_POINT ( 'NONE',  ( -13.14518615778179544, 35.98945312608393721, 0.000000000000000000 ) ) ;
#5624=CARTESIAN_POINT ( 'NONE',  ( -8.049105076161786076E-16, 31.62382812608393579, -13.14518615778179544 ) ) ;
#5630=CARTESIAN_POINT ( 'NONE',  ( 0.000000000000000000, 40.99999999999999289, -13.57481594606304576 ) ) ;
#5639=ORIENTED_EDGE ( 'NONE', *, *, #22680, .T. ) ;
#5643=CARTESIAN_POINT ( 'NONE',  ( -13.57481594606304398, 40.25585937499999289, 5.622872871577880183 ) ) ;
#5655=CARTESIAN_POINT ( 'NONE',  ( 13.57481594606304931, 39.75976562499999289, 5.622872871577869525 ) ) ;
#5656=CARTESIAN_POINT ( 'NONE',  ( -5.622872871577873077, 32.51679687716787726, 13.57481594606304753 ) ) ;
#5669=CARTESIAN_POINT ( 'NONE',  ( 1.662435489736055892E-15, 40.99999999999999289, 13.57481594606304576 ) ) ;
#5679=CARTESIAN_POINT ( 'NONE',  ( 13.57481594606304576, 40.60312499999999858, -1.662435489736055892E-15 ) ) ;
#5681=CARTESIAN_POINT ( 'NONE',  ( 9.295050272127046043, 33.90585937608393152, -9.295050272127046043 ) ) ;
#5718=PRODUCT_CONTEXT ( 'NONE', #20626, 'mechanical' ) ;
#5741=CARTESIAN_POINT ( 'NONE',  ( 13.14518615778179722, 38.61875000108392442, -5.444914386472297529 ) ) ;
#5746=DIRECTION ( 'NONE',  ( 0.000000000000000000, 1.000000000000000000, 0.000000000000000000 ) ) ;
#5749=CARTESIAN_POINT ( 'NONE',  ( -8.049105076161786076E-16, 33.40976562608393863, -13.14518615778179544 ) ) ;
#5754=CARTESIAN_POINT ( 'NONE',  ( 5.622872871577742515, 38.96601562716787015, 13.57481594606318076 ) ) ;
#5761=CARTESIAN_POINT ( 'NONE',  ( -9.295050272127046043, 31.72304687608393081, -9.295050272127046043 ) ) ;
#5762=AXIS2_PLACEMENT_3D ( 'NONE', #19461, #28158, #23877 ) ;
#5763=ORIENTED_EDGE ( 'NONE', *, *, #6347, .F. ) ;
#5775=ORIENTED_EDGE ( 'NONE', *, *, #10019, .T. ) ;
#5793=CARTESIAN_POINT ( 'NONE',  ( -9.598844408820454532, 37.22968750216787726, 9.598844408820459861 ) ) ;
#5795=CARTESIAN_POINT ( 'NONE',  ( 9.598844408820456309, 39.11484374999999858, -9.598844408820458085 ) ) ;
#5796=CARTESIAN_POINT ( 'NONE',  ( -8.049105076161786076E-16, 40.35507812608393152, -13.14518615778179544 ) ) ;
#5826=( BOUNDED_CURVE ( )  B_SPLINE_CURVE ( 2, ( #17493, #4533, #8802, #17067, #12912, #10786, #19776, #19636, #14921 ),
 .UNSPECIFIED., .F., .F. ) 
 B_SPLINE_CURVE_WITH_KNOTS ( ( 3, 2, 2, 2, 3 ),
 ( 0.6458333333333333703, 0.6562500000000000000, 0.6666666666666665186, 0.6770833333333332593, 0.6874999999999997780 ),
 .UNSPECIFIED. ) 
 CURVE ( )  GEOMETRIC_REPRESENTATION_ITEM ( )  RATIONAL_B_SPLINE_CURVE ( ( 1.000000000000000000, 0.9238795325112867385, 1.000000000000000000, 0.9238795325112867385, 1.000000000000000000, 0.9238795325112867385, 1.000000000000000000, 0.9238795325112884038, 0.9999999999999983347 ) ) 
 REPRESENTATION_ITEM ( '' )  );
#5828=CARTESIAN_POINT ( 'NONE',  ( 13.57481594606304576, 33.45937499999999432, -1.662435489736055892E-15 ) ) ;
#5833=CARTESIAN_POINT ( 'NONE',  ( -5.444914386472297529, 40.60312500108393863, -13.14518615778179900 ) ) ;
#5834=CARTESIAN_POINT ( 'NONE',  ( 13.57481594606304931, 39.06523437716786873, 5.622872871577869525 ) ) ;
#5854=DIRECTION ( 'NONE',  ( -0.000000000000000000, -1.000000000000000000, -0.000000000000000000 ) ) ;
#5870=( BOUNDED_CURVE ( )  B_SPLINE_CURVE ( 2, ( #25343, #12766, #7819, #14357, #5828, #10076, #10633, #6923, #9070 ),
 .UNSPECIFIED., .F., .F. ) 
 B_SPLINE_CURVE_WITH_KNOTS ( ( 3, 2, 2, 2, 3 ),
 ( 0.7708333333333333703, 0.7812500000000000000, 0.7916666666666665186, 0.8020833333333332593, 0.8124999999999998890 ),
 .UNSPECIFIED. ) 
 CURVE ( )  GEOMETRIC_REPRESENTATION_ITEM ( )  RATIONAL_B_SPLINE_CURVE ( ( 1.000000000000000000, 0.9238795325112867385, 1.000000000000000000, 0.9238795325112867385, 1.000000000000000000, 0.9238795325112867385, 1.000000000000000000, 0.9238795325112875156, 0.9999999999999992228 ) ) 
 REPRESENTATION_ITEM ( '' )  );
#5878=CARTESIAN_POINT ( 'NONE',  ( -8.049105076161786076E-16, 39.56132812608393579, -13.14518615778179544 ) ) ;
#5895=CARTESIAN_POINT ( 'NONE',  ( 13.57481594606304576, 39.11484375216787157, -1.662435489736055892E-15 ) ) ;
#5900=DIRECTION ( 'NONE',  ( 1.000000000000000000, 0.000000000000000000, 0.000000000000000000 ) ) ;
#5909=CARTESIAN_POINT ( 'NONE',  ( 5.622872871577878406, 34.89804687499999147, 13.57481594606304398 ) ) ;
#5930=CARTESIAN_POINT ( 'NONE',  ( -9.598844408820458085, 40.10703124999999147, -9.598844408820458085 ) ) ;
#5931=CARTESIAN_POINT ( 'NONE',  ( -9.598844408820454532, 32.46718750216787441, 9.598844408820459861 ) ) ;
#5940=DIRECTION ( 'NONE',  ( 0.000000000000000000, 0.000000000000000000, -1.000000000000000000 ) ) ;
#5946=CARTESIAN_POINT ( 'NONE',  ( 0.000000000000000000, 40.99999999999999289, -15.57481594606304576 ) ) ;
#5964=ORIENTED_EDGE ( 'NONE', *, *, #11204, .F. ) ;
#5966=CARTESIAN_POINT ( 'NONE',  ( 5.444914386472297529, 38.91640625108393436, -13.14518615778179900 ) ) ;
#5967=CARTESIAN_POINT ( 'NONE',  ( 13.57481594606304753, 39.95820312716787726, -5.622872871577873077 ) ) ;
#5985=( BOUNDED_SURFACE ( )  B_SPLINE_SURFACE ( 1, 2, ( 
 ( #23630, #19345, #18793, #5833, #23079, #16789, #16654, #1698, #28048, #25349, #12211, #14501, #8515, #19207, #27635, #23218, #3694, #25488, #20940, #12357, #21075, #3826, #1564, #14635, #27772, #10500, #4106, #10355, #8371, #17055, #23353, #12772, #25759, #18927, #21489, #8095, #23490, #5966, #12487, #1970, #8230, #16921, #25621, #6103, #14770, #10638, #17199, #19763, #2108, #9076, #2396, #13469, #8653, #394, #108, #6646, #26329, #15474, #17910, #24189, #28185, #13330, #21776, #22056, #2255, #26621, #19626, #8790, #10917, #6931, #22195, #2674, #21632, #15048, #19911, #15332, #10775, #23766, #11054, #15624, #11335, #23904, #13182, #24048, #8933, #4384, #4242, #12902, #6789, #26475, #19487, #17771, #4668, #24326, #4523, #2530, #17344, #26040, #6511, #535, #9217, #21921, #247, #17622, #4810, #11192, #20056, #15186, #13041, #17481, #26180, #22624, #3366, #3232, #26761, #11900, #5093, #4955, #13899, #11762, #16042, #18622, #16190, #11615, #5518, #2945, #16336, #20761, #26905, #9355, #15898, #27192, #5377, #7203, #9636, #5233, #7351, #680, #20486, #22767, #27046, #18048, #24896, #7068, #967, #22339, #1109, #3095, #14185, #24615, #20624, #20340, #24752, #18341, #7494, #9908, #14046, #20195, #9776, #13755, #18484, #22480, #15763, #827, #9494, #18194, #7643, #22903, #12037, #13616, #24470, #25036, #1245, #2809, #11478, #14598, #27870, #6203, #7918, #25450, #18884, #21174, #16614 ),
 ( #27734, #1796, #8054, #19021, #12173, #20903, #25167, #12732, #21456, #27593, #23316, #16749, #12588, #14732, #21312, #19169, #10461, #1385, #5930, #3789, #23588, #23452, #18757, #3930, #25307, #5655, #12447, #1654, #10313, #10603, #8194, #3654, #25720, #23180, #8333, #1934, #16884, #10046, #5795, #17017, #25583, #27460, #6066, #14873, #4070, #14461, #27326, #7785, #16472, #12317, #14320, #21038, #23041, #1522, #3512, #10174, #10739, #72, #25865, #10880, #24011, #17586, #19870, #6609, #24152, #4629, #19589, #11154, #13287, #28148, #26291, #15010, #19726, #2637, #8615, #355, #15149, #13146, #4205, #4345, #2216, #22159, #11013, #2069, #211, #19449, #23731, #13001, #19310, #28010, #17303, #8753, #6336, #17445, #4489, #6753, #9042, #15294, #22016, #2493, #26144, #17734, #26436, #26003, #15437, #12864, #8896, #8475, #6474, #6895, #23867, #21883, #21594, #21740, #2358, #17164, #15582, #24290, #4771, #13431, #26871, #9741, #4918, #24859, #24576, #2911, #22588, #11723, #14150, #20449, #24430, #9602, #18013, #18303, #26724, #22869, #15866, #5058, #7169, #3196, #18450, #27156, #17874, #11299, #16153, #11581, #26580, #20020, #7317, #11867, #7609, #20161, #9457, #20301, #5198, #643, #500, #9181, #3057, #22729, #7029, #14006, #931, #20589, #787, #27011, #13579, #22302, #15726, #25000, #5480, #18159, #16006, #24720, #5340, #7458, #1072, #16299, #2777, #11441, #13863, #9316, #13722 ) ),
 .UNSPECIFIED., .F., .F., .F. ) 
 B_SPLINE_SURFACE_WITH_KNOTS ( ( 2, 2 ),
 ( 3, 2, 2, 2, 2, 2, 2, 2, 2, 2, 2, 2, 2, 2, 2, 2, 2, 2, 2, 2, 2, 2, 2, 2, 2, 2, 2, 2, 2, 2, 2, 2, 2, 2, 2, 2, 2, 2, 2, 2, 2, 2, 2, 2, 2, 2, 2, 2, 2, 2, 2, 2, 2, 2, 2, 2, 2, 2, 2, 2, 2, 2, 2, 2, 2, 2, 2, 2, 2, 2, 2, 2, 2, 2, 2, 2, 2, 2, 2, 2, 2, 2, 2, 2, 2, 2, 2, 2, 2, 2, 2, 3 ),
 ( 0.000000000000000000, 1.000000000000000000 ),
 ( 0.000000000000000000, 0.01041666666666666609, 0.02083333333333333218, 0.03125000000000000000, 0.04166666666666666435, 0.05208333333333333565, 0.06250000000000000000, 0.07291666666666667129, 0.08333333333333332871, 0.09375000000000000000, 0.1041666666666666713, 0.1145833333333333287, 0.1250000000000000000, 0.1354166666666666574, 0.1458333333333333426, 0.1562500000000000000, 0.1666666666666666574, 0.1770833333333333426, 0.1875000000000000000, 0.1979166666666666574, 0.2083333333333333426, 0.2187500000000000000, 0.2291666666666666574, 0.2395833333333333426, 0.2500000000000000000, 0.2604166666666666852, 0.2708333333333333148, 0.2812500000000000000, 0.2916666666666666852, 0.3020833333333333148, 0.3125000000000000000, 0.3229166666666666852, 0.3333333333333333148, 0.3437500000000000000, 0.3541666666666666852, 0.3645833333333333148, 0.3750000000000000000, 0.3854166666666666852, 0.3958333333333333148, 0.4062500000000000000, 0.4166666666666666852, 0.4270833333333333148, 0.4375000000000000000, 0.4479166666666666852, 0.4583333333333333148, 0.4687500000000000000, 0.4791666666666666852, 0.4895833333333333148, 0.5000000000000000000, 0.5104166666666666297, 0.5208333333333333703, 0.5312500000000000000, 0.5416666666666666297, 0.5520833333333333703, 0.5625000000000000000, 0.5729166666666666297, 0.5833333333333333703, 0.5937500000000000000, 0.6041666666666666297, 0.6145833333333333703, 0.6250000000000000000, 0.6354166666666666297, 0.6458333333333333703, 0.6562500000000000000, 0.6666666666666666297, 0.6770833333333333703, 0.6875000000000000000, 0.6979166666666666297, 0.7083333333333333703, 0.7187500000000000000, 0.7291666666666666297, 0.7395833333333333703, 0.7500000000000000000, 0.7604166666666666297, 0.7708333333333333703, 0.7812500000000000000, 0.7916666666666666297, 0.8020833333333333703, 0.8125000000000000000, 0.8229166666666666297, 0.8333333333333333703, 0.8437500000000000000, 0.8541666666666666297, 0.8645833333333333703, 0.8750000000000000000, 0.8854166666666666297, 0.8958333333333333703, 0.9062500000000000000, 0.9166666666666666297, 0.9270833333333333703, 0.9375000000000000000, 0.9448586968893691873 ),
 .UNSPECIFIED. ) 
 GEOMETRIC_REPRESENTATION_ITEM ( )  RATIONAL_B_SPLINE_SURFACE ( (
 ( 1.000000000000000000, 0.9238795325112867385, 1.000000000000000000, 0.9238795325112867385, 1.000000000000000000, 0.9238795325112867385, 1.000000000000000000, 0.9238795325112867385, 1.000000000000000000, 0.9238795325112867385, 1.000000000000000000, 0.9238795325112867385, 1.000000000000000000, 0.9238795325112867385, 1.000000000000000000, 0.9238795325112867385, 1.000000000000000000, 0.9238795325112867385, 1.000000000000000000, 0.9238795325112867385, 1.000000000000000000, 0.9238795325112867385, 1.000000000000000000, 0.9238795325112867385, 1.000000000000000000, 0.9238795325112867385, 1.000000000000000000, 0.9238795325112867385, 1.000000000000000000, 0.9238795325112867385, 1.000000000000000000, 0.9238795325112867385, 1.000000000000000000, 0.9238795325112867385, 1.000000000000000000, 0.9238795325112867385, 1.000000000000000000, 0.9238795325112867385, 1.000000000000000000, 0.9238795325112867385, 1.000000000000000000, 0.9238795325112867385, 1.000000000000000000, 0.9238795325112867385, 1.000000000000000000, 0.9238795325112867385, 1.000000000000000000, 0.9238795325112867385, 1.000000000000000000, 0.9238795325112867385, 1.000000000000000000, 0.9238795325112867385, 1.000000000000000000, 0.9238795325112867385, 1.000000000000000000, 0.9238795325112867385, 1.000000000000000000, 0.9238795325112867385, 1.000000000000000000, 0.9238795325112867385, 1.000000000000000000, 0.9238795325112867385, 1.000000000000000000, 0.9238795325112867385, 1.000000000000000000, 0.9238795325112867385, 1.000000000000000000, 0.9238795325112867385, 1.000000000000000000, 0.9238795325112867385, 1.000000000000000000, 0.9238795325112867385, 1.000000000000000000, 0.9238795325112867385, 1.000000000000000000, 0.9238795325112867385, 1.000000000000000000, 0.9238795325112867385, 1.000000000000000000, 0.9238795325112867385, 1.000000000000000000, 0.9238795325112867385, 1.000000000000000000, 0.9238795325112867385, 1.000000000000000000, 0.9238795325112867385, 1.000000000000000000, 0.9238795325112867385, 1.000000000000000000, 0.9238795325112867385, 1.000000000000000000, 0.9238795325112867385, 1.000000000000000000, 0.9238795325112867385, 1.000000000000000000, 0.9238795325112867385, 1.000000000000000000, 0.9238795325112867385, 1.000000000000000000, 0.9238795325112867385, 1.000000000000000000, 0.9238795325112867385, 1.000000000000000000, 0.9238795325112867385, 1.000000000000000000, 0.9238795325112867385, 1.000000000000000000, 0.9238795325112867385, 1.000000000000000000, 0.9238795325112867385, 1.000000000000000000, 0.9238795325112867385, 1.000000000000000000, 0.9238795325112867385, 1.000000000000000000, 0.9238795325112867385, 1.000000000000000000, 0.9238795325112867385, 1.000000000000000000, 0.9238795325112867385, 1.000000000000000000, 0.9238795325112867385, 1.000000000000000000, 0.9238795325112867385, 1.000000000000000000, 0.9238795325112867385, 1.000000000000000000, 0.9238795325112867385, 1.000000000000000000, 0.9238795325112867385, 1.000000000000000000, 0.9238795325112867385, 1.000000000000000000, 0.9238795325112867385, 1.000000000000000000, 0.9238795325112867385, 1.000000000000000000, 0.9238795325112867385, 1.000000000000000000, 0.9238795325112867385, 1.000000000000000000, 0.9238795325112867385, 1.000000000000000000, 0.9238795325112867385, 1.000000000000000000, 0.9238795325112867385, 1.000000000000000000, 0.9238795325112867385, 1.000000000000000000, 0.9238795325112867385, 1.000000000000000000, 0.9238795325112867385, 1.000000000000000000, 0.9238795325112867385, 1.000000000000000000, 0.9238795325112867385, 1.000000000000000000, 0.9238795325112867385, 1.000000000000000000, 0.9238795325112867385, 1.000000000000000000, 0.9238795325112867385, 1.000000000000000000, 0.9238795325112867385, 1.000000000000000000, 0.9238795325112867385, 1.000000000000000000, 0.9238795325112867385, 1.000000000000000000, 0.9238795325112867385, 1.000000000000000000, 0.9238795325112867385, 1.000000000000000000, 0.9238795325112867385, 1.000000000000000000, 0.9238795325112867385, 1.000000000000000000, 0.9238795325112867385, 1.000000000000000000, 0.9238795325112867385, 1.000000000000000000, 0.9462258450566536361, 0.9684275698016389100),
 ( 1.000000000000000000, 0.9238795325112867385, 1.000000000000000000, 0.9238795325112867385, 1.000000000000000000, 0.9238795325112867385, 1.000000000000000000, 0.9238795325112867385, 1.000000000000000000, 0.9238795325112867385, 1.000000000000000000, 0.9238795325112867385, 1.000000000000000000, 0.9238795325112867385, 1.000000000000000000, 0.9238795325112867385, 1.000000000000000000, 0.9238795325112867385, 1.000000000000000000, 0.9238795325112867385, 1.000000000000000000, 0.9238795325112867385, 1.000000000000000000, 0.9238795325112867385, 1.000000000000000000, 0.9238795325112867385, 1.000000000000000000, 0.9238795325112867385, 1.000000000000000000, 0.9238795325112867385, 1.000000000000000000, 0.9238795325112867385, 1.000000000000000000, 0.9238795325112867385, 1.000000000000000000, 0.9238795325112867385, 1.000000000000000000, 0.9238795325112867385, 1.000000000000000000, 0.9238795325112867385, 1.000000000000000000, 0.9238795325112867385, 1.000000000000000000, 0.9238795325112867385, 1.000000000000000000, 0.9238795325112867385, 1.000000000000000000, 0.9238795325112867385, 1.000000000000000000, 0.9238795325112867385, 1.000000000000000000, 0.9238795325112867385, 1.000000000000000000, 0.9238795325112867385, 1.000000000000000000, 0.9238795325112867385, 1.000000000000000000, 0.9238795325112867385, 1.000000000000000000, 0.9238795325112867385, 1.000000000000000000, 0.9238795325112867385, 1.000000000000000000, 0.9238795325112867385, 1.000000000000000000, 0.9238795325112867385, 1.000000000000000000, 0.9238795325112867385, 1.000000000000000000, 0.9238795325112867385, 1.000000000000000000, 0.9238795325112867385, 1.000000000000000000, 0.9238795325112867385, 1.000000000000000000, 0.9238795325112867385, 1.000000000000000000, 0.9238795325112867385, 1.000000000000000000, 0.9238795325112867385, 1.000000000000000000, 0.9238795325112867385, 1.000000000000000000, 0.9238795325112867385, 1.000000000000000000, 0.9238795325112867385, 1.000000000000000000, 0.9238795325112867385, 1.000000000000000000, 0.9238795325112867385, 1.000000000000000000, 0.9238795325112867385, 1.000000000000000000, 0.9238795325112867385, 1.000000000000000000, 0.9238795325112867385, 1.000000000000000000, 0.9238795325112867385, 1.000000000000000000, 0.9238795325112867385, 1.000000000000000000, 0.9238795325112867385, 1.000000000000000000, 0.9238795325112867385, 1.000000000000000000, 0.9238795325112867385, 1.000000000000000000, 0.9238795325112867385, 1.000000000000000000, 0.9238795325112867385, 1.000000000000000000, 0.9238795325112867385, 1.000000000000000000, 0.9238795325112867385, 1.000000000000000000, 0.9238795325112867385, 1.000000000000000000, 0.9238795325112867385, 1.000000000000000000, 0.9238795325112867385, 1.000000000000000000, 0.9238795325112867385, 1.000000000000000000, 0.9238795325112867385, 1.000000000000000000, 0.9238795325112867385, 1.000000000000000000, 0.9238795325112867385, 1.000000000000000000, 0.9238795325112867385, 1.000000000000000000, 0.9238795325112867385, 1.000000000000000000, 0.9238795325112867385, 1.000000000000000000, 0.9238795325112867385, 1.000000000000000000, 0.9238795325112867385, 1.000000000000000000, 0.9238795325112867385, 1.000000000000000000, 0.9238795325112867385, 1.000000000000000000, 0.9238795325112867385, 1.000000000000000000, 0.9238795325112867385, 1.000000000000000000, 0.9238795325112867385, 1.000000000000000000, 0.9238795325112867385, 1.000000000000000000, 0.9238795325112867385, 1.000000000000000000, 0.9238795325112867385, 1.000000000000000000, 0.9238795325112867385, 1.000000000000000000, 0.9238795325112867385, 1.000000000000000000, 0.9238795325112867385, 1.000000000000000000, 0.9238795325112867385, 1.000000000000000000, 0.9238795325112867385, 1.000000000000000000, 0.9238795325112867385, 1.000000000000000000, 0.9238795325112867385, 1.000000000000000000, 0.9238795325112867385, 1.000000000000000000, 0.9238795325112867385, 1.000000000000000000, 0.9238795325112867385, 1.000000000000000000, 0.9238795325112867385, 1.000000000000000000, 0.9238795325112867385, 1.000000000000000000, 0.9238795325112867385, 1.000000000000000000, 0.9462258450566536361, 0.9684275698016389100) ) ) 
 REPRESENTATION_ITEM ( '' )  SURFACE ( )  );
#5986=CARTESIAN_POINT ( 'NONE',  ( 13.14518615778179900, 40.20625000108393010, -5.444914386472297529 ) ) ;
#6003=ORIENTED_EDGE ( 'NONE', *, *, #22404, .T. ) ;
#6024=CARTESIAN_POINT ( 'NONE',  ( 5.444914386472302859, 33.06250000108393294, 13.14518615778179189 ) ) ;
#6031=CARTESIAN_POINT ( 'NONE',  ( -9.295050272127044266, 32.91367187608393152, 9.295050272127047819 ) ) ;
#6032=( BOUNDED_SURFACE ( )  B_SPLINE_SURFACE ( 1, 2, ( 
 ( #26060, #23509, #8672, #13059, #3988, #21653, #12504, #5986, #19226, #25507, #2128, #14652, #14930, #15206, #10793, #25923, #17364, #19507, #8387, #6528, #23371, #21376, #10934, #8114, #19084, #25778, #21233, #6256, #2275, #1716, #8249, #23926, #27654, #10377, #18138, #16808, #12790, #4405, #23650, #12651, #14786, #4125, #6397, #27791, #16937, #25637, #6120, #21508, #23784, #1989, #10655, #1854, #19363, #28066, #8532, #17218, #8812, #15351, #2555, #13778, #24491, #19931, #4976, #9098, #26351, #557, #26495, #24637, #15647, #24210, #7230, #8954, #11499, #22500, #21939, #9374, #18070, #6952, #26785, #269, #26202, #2965, #24345, #20216, #15921, #17644, #17793, #11215, #13497, #6810, #19644, #127, #5113, #17502, #6666, #414, #4836, #24067, #22217, #15498, #2695, #11356, #19787, #13641, #4543, #20079, #4689, #13205, #9239, #2416, #11075, #13349, #22078, #17931, #22356, #26641, #7088, #15788, #2831, #701, #12574, #23438, #25059, #23577, #9521, #10449, #24775, #21301, #1267, #26929, #9931, #5256, #991, #7372, #5681, #25194, #1131, #9800, #27069, #11640, #22648, #3117, #14069, #3915, #27859, #11926, #16067, #25709, #1783, #17005, #16215, #22929, #20508, #16359, #3390, #11785, #20786, #14860, #19156, #22789, #18220, #18506, #8319, #5545, #12061, #20363, #6190, #7520, #848, #13920, #27212, #14209, #9659, #18361, #24916, #5400, #3259, #20648, #7667, #18646, #27351, #7809, #16499 ),
 ( #14720, #4614, #11140, #12853, #2202, #23854, #26132, #21581, #6883, #12719, #9031, #19856, #343, #25992, #8459, #19714, #23718, #19576, #17572, #2479, #26278, #10863, #13133, #25850, #17433, #19435, #6739, #15424, #14998, #12989, #24137, #6323, #21729, #60, #17723, #28134, #13273, #26425, #8602, #8882, #17148, #10591, #4332, #1923, #22003, #19298, #8740, #15570, #4057, #2345, #21445, #27998, #15135, #4194, #2058, #6461, #10727, #17290, #6598, #15281, #24000, #4476, #21868, #11001, #199, #13991, #24278, #26566, #917, #18435, #9445, #22717, #22431, #20150, #11430, #15855, #3041, #22145, #11287, #9588, #27143, #2899, #11711, #772, #24564, #4905, #18002, #13567, #11855, #629, #13419, #20008, #7159, #7595, #18292, #5045, #26998, #13710, #2766, #5186, #11569, #1060, #20286, #9304, #20577, #22290, #16141, #4759, #7019, #3185, #9730, #18145, #2625, #26710, #488, #9170, #26859, #24849, #17862, #7305, #15992, #24706, #13849, #22574, #15714, #24416, #20436, #7445, #5327, #10001, #20718, #3747, #7735, #3609, #1614, #14688, #10272, #23132, #25407, #9869, #1474, #3463, #18981, #27690, #27279, #25258, #8153, #18576, #5749, #12268, #1201, #16846, #25544, #16425, #12408, #6024, #25121, #23407, #21128, #16567, #3882, #12543, #24986, #14417, #20994, #14275, #5609, #21269, #1753, #27410, #10419, #10131, #16709, #22993, #3323, #19125, #18843, #27832, #12128, #16285, #20855, #18708, #1337 ) ),
 .UNSPECIFIED., .F., .F., .F. ) 
 B_SPLINE_SURFACE_WITH_KNOTS ( ( 2, 2 ),
 ( 3, 2, 2, 2, 2, 2, 2, 2, 2, 2, 2, 2, 2, 2, 2, 2, 2, 2, 2, 2, 2, 2, 2, 2, 2, 2, 2, 2, 2, 2, 2, 2, 2, 2, 2, 2, 2, 2, 2, 2, 2, 2, 2, 2, 2, 2, 2, 2, 2, 2, 2, 2, 2, 2, 2, 2, 2, 2, 2, 2, 2, 2, 2, 2, 2, 2, 2, 2, 2, 2, 2, 2, 2, 2, 2, 2, 2, 2, 2, 2, 2, 2, 2, 2, 2, 2, 2, 2, 2, 2, 2, 3 ),
 ( 0.000000000000000000, 1.000000000000000000 ),
 ( 0.000000000000000000, 0.01041666666666666609, 0.02083333333333333218, 0.03125000000000000000, 0.04166666666666666435, 0.05208333333333333565, 0.06250000000000000000, 0.07291666666666667129, 0.08333333333333332871, 0.09375000000000000000, 0.1041666666666666713, 0.1145833333333333287, 0.1250000000000000000, 0.1354166666666666574, 0.1458333333333333426, 0.1562500000000000000, 0.1666666666666666574, 0.1770833333333333426, 0.1875000000000000000, 0.1979166666666666574, 0.2083333333333333426, 0.2187500000000000000, 0.2291666666666666574, 0.2395833333333333426, 0.2500000000000000000, 0.2604166666666666852, 0.2708333333333333148, 0.2812500000000000000, 0.2916666666666666852, 0.3020833333333333148, 0.3125000000000000000, 0.3229166666666666852, 0.3333333333333333148, 0.3437500000000000000, 0.3541666666666666852, 0.3645833333333333148, 0.3750000000000000000, 0.3854166666666666852, 0.3958333333333333148, 0.4062500000000000000, 0.4166666666666666852, 0.4270833333333333148, 0.4375000000000000000, 0.4479166666666666852, 0.4583333333333333148, 0.4687500000000000000, 0.4791666666666666852, 0.4895833333333333148, 0.5000000000000000000, 0.5104166666666666297, 0.5208333333333333703, 0.5312500000000000000, 0.5416666666666666297, 0.5520833333333333703, 0.5625000000000000000, 0.5729166666666666297, 0.5833333333333333703, 0.5937500000000000000, 0.6041666666666666297, 0.6145833333333333703, 0.6250000000000000000, 0.6354166666666666297, 0.6458333333333333703, 0.6562500000000000000, 0.6666666666666666297, 0.6770833333333333703, 0.6875000000000000000, 0.6979166666666666297, 0.7083333333333333703, 0.7187500000000000000, 0.7291666666666666297, 0.7395833333333333703, 0.7500000000000000000, 0.7604166666666666297, 0.7708333333333333703, 0.7812500000000000000, 0.7916666666666666297, 0.8020833333333333703, 0.8125000000000000000, 0.8229166666666666297, 0.8333333333333333703, 0.8437500000000000000, 0.8541666666666666297, 0.8645833333333333703, 0.8750000000000000000, 0.8854166666666666297, 0.8958333333333333703, 0.9062500000000000000, 0.9166666666666666297, 0.9270833333333333703, 0.9375000000000000000, 0.9448587001587775980 ),
 .UNSPECIFIED. ) 
 GEOMETRIC_REPRESENTATION_ITEM ( )  RATIONAL_B_SPLINE_SURFACE ( (
 ( 1.000000000000000000, 0.9238795325112867385, 1.000000000000000000, 0.9238795325112867385, 1.000000000000000000, 0.9238795325112867385, 1.000000000000000000, 0.9238795325112867385, 1.000000000000000000, 0.9238795325112867385, 1.000000000000000000, 0.9238795325112867385, 1.000000000000000000, 0.9238795325112867385, 1.000000000000000000, 0.9238795325112867385, 1.000000000000000000, 0.9238795325112867385, 1.000000000000000000, 0.9238795325112867385, 1.000000000000000000, 0.9238795325112867385, 1.000000000000000000, 0.9238795325112867385, 1.000000000000000000, 0.9238795325112867385, 1.000000000000000000, 0.9238795325112867385, 1.000000000000000000, 0.9238795325112867385, 1.000000000000000000, 0.9238795325112867385, 1.000000000000000000, 0.9238795325112867385, 1.000000000000000000, 0.9238795325112867385, 1.000000000000000000, 0.9238795325112867385, 1.000000000000000000, 0.9238795325112867385, 1.000000000000000000, 0.9238795325112867385, 1.000000000000000000, 0.9238795325112867385, 1.000000000000000000, 0.9238795325112867385, 1.000000000000000000, 0.9238795325112867385, 1.000000000000000000, 0.9238795325112867385, 1.000000000000000000, 0.9238795325112867385, 1.000000000000000000, 0.9238795325112867385, 1.000000000000000000, 0.9238795325112867385, 1.000000000000000000, 0.9238795325112867385, 1.000000000000000000, 0.9238795325112867385, 1.000000000000000000, 0.9238795325112867385, 1.000000000000000000, 0.9238795325112867385, 1.000000000000000000, 0.9238795325112867385, 1.000000000000000000, 0.9238795325112867385, 1.000000000000000000, 0.9238795325112867385, 1.000000000000000000, 0.9238795325112867385, 1.000000000000000000, 0.9238795325112867385, 1.000000000000000000, 0.9238795325112867385, 1.000000000000000000, 0.9238795325112867385, 1.000000000000000000, 0.9238795325112867385, 1.000000000000000000, 0.9238795325112867385, 1.000000000000000000, 0.9238795325112867385, 1.000000000000000000, 0.9238795325112867385, 1.000000000000000000, 0.9238795325112867385, 1.000000000000000000, 0.9238795325112867385, 1.000000000000000000, 0.9238795325112867385, 1.000000000000000000, 0.9238795325112867385, 1.000000000000000000, 0.9238795325112867385, 1.000000000000000000, 0.9238795325112867385, 1.000000000000000000, 0.9238795325112867385, 1.000000000000000000, 0.9238795325112867385, 1.000000000000000000, 0.9238795325112867385, 1.000000000000000000, 0.9238795325112867385, 1.000000000000000000, 0.9238795325112867385, 1.000000000000000000, 0.9238795325112867385, 1.000000000000000000, 0.9238795325112867385, 1.000000000000000000, 0.9238795325112867385, 1.000000000000000000, 0.9238795325112867385, 1.000000000000000000, 0.9238795325112867385, 1.000000000000000000, 0.9238795325112867385, 1.000000000000000000, 0.9238795325112867385, 1.000000000000000000, 0.9238795325112867385, 1.000000000000000000, 0.9238795325112867385, 1.000000000000000000, 0.9238795325112867385, 1.000000000000000000, 0.9238795325112867385, 1.000000000000000000, 0.9238795325112867385, 1.000000000000000000, 0.9238795325112867385, 1.000000000000000000, 0.9238795325112867385, 1.000000000000000000, 0.9238795325112867385, 1.000000000000000000, 0.9238795325112867385, 1.000000000000000000, 0.9238795325112867385, 1.000000000000000000, 0.9238795325112867385, 1.000000000000000000, 0.9238795325112867385, 1.000000000000000000, 0.9238795325112867385, 1.000000000000000000, 0.9238795325112867385, 1.000000000000000000, 0.9238795325112867385, 1.000000000000000000, 0.9238795325112867385, 1.000000000000000000, 0.9238795325112867385, 1.000000000000000000, 0.9238795325112867385, 1.000000000000000000, 0.9238795325112867385, 1.000000000000000000, 0.9238795325112867385, 1.000000000000000000, 0.9238795325112867385, 1.000000000000000000, 0.9238795325112867385, 1.000000000000000000, 0.9238795325112867385, 1.000000000000000000, 0.9238795325112867385, 1.000000000000000000, 0.9238795325112867385, 1.000000000000000000, 0.9238795325112867385, 1.000000000000000000, 0.9238795325112867385, 1.000000000000000000, 0.9238795325112867385, 1.000000000000000000, 0.9238795325112867385, 1.000000000000000000, 0.9462258211652395667, 0.9684275895297407288),
 ( 1.000000000000000000, 0.9238795325112867385, 1.000000000000000000, 0.9238795325112867385, 1.000000000000000000, 0.9238795325112867385, 1.000000000000000000, 0.9238795325112867385, 1.000000000000000000, 0.9238795325112867385, 1.000000000000000000, 0.9238795325112867385, 1.000000000000000000, 0.9238795325112867385, 1.000000000000000000, 0.9238795325112867385, 1.000000000000000000, 0.9238795325112867385, 1.000000000000000000, 0.9238795325112867385, 1.000000000000000000, 0.9238795325112867385, 1.000000000000000000, 0.9238795325112867385, 1.000000000000000000, 0.9238795325112867385, 1.000000000000000000, 0.9238795325112867385, 1.000000000000000000, 0.9238795325112867385, 1.000000000000000000, 0.9238795325112867385, 1.000000000000000000, 0.9238795325112867385, 1.000000000000000000, 0.9238795325112867385, 1.000000000000000000, 0.9238795325112867385, 1.000000000000000000, 0.9238795325112867385, 1.000000000000000000, 0.9238795325112867385, 1.000000000000000000, 0.9238795325112867385, 1.000000000000000000, 0.9238795325112867385, 1.000000000000000000, 0.9238795325112867385, 1.000000000000000000, 0.9238795325112867385, 1.000000000000000000, 0.9238795325112867385, 1.000000000000000000, 0.9238795325112867385, 1.000000000000000000, 0.9238795325112867385, 1.000000000000000000, 0.9238795325112867385, 1.000000000000000000, 0.9238795325112867385, 1.000000000000000000, 0.9238795325112867385, 1.000000000000000000, 0.9238795325112867385, 1.000000000000000000, 0.9238795325112867385, 1.000000000000000000, 0.9238795325112867385, 1.000000000000000000, 0.9238795325112867385, 1.000000000000000000, 0.9238795325112867385, 1.000000000000000000, 0.9238795325112867385, 1.000000000000000000, 0.9238795325112867385, 1.000000000000000000, 0.9238795325112867385, 1.000000000000000000, 0.9238795325112867385, 1.000000000000000000, 0.9238795325112867385, 1.000000000000000000, 0.9238795325112867385, 1.000000000000000000, 0.9238795325112867385, 1.000000000000000000, 0.9238795325112867385, 1.000000000000000000, 0.9238795325112867385, 1.000000000000000000, 0.9238795325112867385, 1.000000000000000000, 0.9238795325112867385, 1.000000000000000000, 0.9238795325112867385, 1.000000000000000000, 0.9238795325112867385, 1.000000000000000000, 0.9238795325112867385, 1.000000000000000000, 0.9238795325112867385, 1.000000000000000000, 0.9238795325112867385, 1.000000000000000000, 0.9238795325112867385, 1.000000000000000000, 0.9238795325112867385, 1.000000000000000000, 0.9238795325112867385, 1.000000000000000000, 0.9238795325112867385, 1.000000000000000000, 0.9238795325112867385, 1.000000000000000000, 0.9238795325112867385, 1.000000000000000000, 0.9238795325112867385, 1.000000000000000000, 0.9238795325112867385, 1.000000000000000000, 0.9238795325112867385, 1.000000000000000000, 0.9238795325112867385, 1.000000000000000000, 0.9238795325112867385, 1.000000000000000000, 0.9238795325112867385, 1.000000000000000000, 0.9238795325112867385, 1.000000000000000000, 0.9238795325112867385, 1.000000000000000000, 0.9238795325112867385, 1.000000000000000000, 0.9238795325112867385, 1.000000000000000000, 0.9238795325112867385, 1.000000000000000000, 0.9238795325112867385, 1.000000000000000000, 0.9238795325112867385, 1.000000000000000000, 0.9238795325112867385, 1.000000000000000000, 0.9238795325112867385, 1.000000000000000000, 0.9238795325112867385, 1.000000000000000000, 0.9238795325112867385, 1.000000000000000000, 0.9238795325112867385, 1.000000000000000000, 0.9238795325112867385, 1.000000000000000000, 0.9238795325112867385, 1.000000000000000000, 0.9238795325112867385, 1.000000000000000000, 0.9238795325112867385, 1.000000000000000000, 0.9238795325112867385, 1.000000000000000000, 0.9238795325112867385, 1.000000000000000000, 0.9238795325112867385, 1.000000000000000000, 0.9238795325112867385, 1.000000000000000000, 0.9238795325112867385, 1.000000000000000000, 0.9238795325112867385, 1.000000000000000000, 0.9238795325112867385, 1.000000000000000000, 0.9238795325112867385, 1.000000000000000000, 0.9238795325112867385, 1.000000000000000000, 0.9238795325112867385, 1.000000000000000000, 0.9462258211652395667, 0.9684275895297407288) ) ) 
 REPRESENTATION_ITEM ( '' )  SURFACE ( )  );
#6042=ORIENTED_EDGE ( 'NONE', *, *, #13151, .F. ) ;
#6061=CARTESIAN_POINT ( 'NONE',  ( 5.444914386472297529, 39.71015625108393010, -13.14518615778179722 ) ) ;
#6066=CARTESIAN_POINT ( 'NONE',  ( 9.598844408820459861, 38.91640624999999432, 9.598844408820456309 ) ) ;
#6067=CARTESIAN_POINT ( 'NONE',  ( -9.295050272127044266, 39.06523437608392868, 9.295050272127047819 ) ) ;
#6076=CARTESIAN_POINT ( 'NONE',  ( -9.598844408820454532, 38.81718750216787583, 9.598844408820459861 ) ) ;
#6084=CARTESIAN_POINT ( 'NONE',  ( -5.622872871577736298, 36.88242187499999858, -13.57481594606318254 ) ) ;
#6103=CARTESIAN_POINT ( 'NONE',  ( 5.444914386472302859, 38.61875000108393152, 13.14518615778179189 ) ) ;
#6104=CARTESIAN_POINT ( 'NONE',  ( 13.57481594606304931, 39.85898437716787157, 5.622872871577869525 ) ) ;
#6120=CARTESIAN_POINT ( 'NONE',  ( -9.295050272127044266, 38.27148437608393294, 9.295050272127047819 ) ) ;
#6123=CARTESIAN_POINT ( 'NONE',  ( -8.312177448680279460E-16, 36.03906250000000000, -13.57481594606304576 ) ) ;
#6133=ORIENTED_EDGE ( 'NONE', *, *, #3595, .T. ) ;
#6141=CARTESIAN_POINT ( 'NONE',  ( -8.312177448680279460E-16, 32.96328125216787441, -13.57481594606304576 ) ) ;
#6143=ORIENTED_EDGE ( 'NONE', *, *, #930, .T. ) ;
#6160=ADVANCED_FACE ( 'NONE', ( #11212 ), #13347, .F. ) ;
#6184=FACE_OUTER_BOUND ( 'NONE', #15691, .T. ) ;
#6190=CARTESIAN_POINT ( 'NONE',  ( 9.295050272127046043, 32.31835937608393294, -9.295050272127046043 ) ) ;
#6196=CARTESIAN_POINT ( 'NONE',  ( -9.295050272127046043, 40.65273437608393436, -9.295050272127046043 ) ) ;
#6203=CARTESIAN_POINT ( 'NONE',  ( -13.14518615778179900, 31.97109375108393436, -5.444914386472297529 ) ) ;
#6204=CARTESIAN_POINT ( 'NONE',  ( 2.493653234604083739E-15, 31.77265625216787370, 13.57481594606304576 ) ) ;
#6224=CARTESIAN_POINT ( 'NONE',  ( -13.57481594606304576, 32.36796875216787583, 0.000000000000000000 ) ) ;
#6242=CARTESIAN_POINT ( 'NONE',  ( -13.57481594606304576, 39.56132812716787583, 5.622872871577880183 ) ) ;
#6256=CARTESIAN_POINT ( 'NONE',  ( 5.444914386472302859, 39.21406250108392300, 13.14518615778179189 ) ) ;
#6262=LINE ( 'NONE', #10800, #10455 ) ;
#6267=VERTEX_POINT ( 'NONE', #2273 ) ;
#6270=EDGE_LOOP ( 'NONE', ( #19724, #4189, #14182, #23384 ) ) ;
#6281=CARTESIAN_POINT ( 'NONE',  ( 5.444914386472302859, 35.24531250108393010, 13.14518615778179189 ) ) ;
#6295=CYLINDRICAL_SURFACE ( 'NONE', #19420, 15.57481594606304576 ) ;
#6300=CARTESIAN_POINT ( 'NONE',  ( -9.295050272127044266, 32.11992187608393579, 9.295050272127047819 ) ) ;
#6308=CARTESIAN_POINT ( 'NONE',  ( 0.000000000000000000, 40.99999999999999289, 0.000000000000000000 ) ) ;
#6311=CYLINDRICAL_SURFACE ( 'NONE', #20320, 13.57481594606304576 ) ;
#6320=VERTEX_POINT ( 'NONE', #7941 ) ;
#6323=CARTESIAN_POINT ( 'NONE',  ( -13.14518615778179189, 39.21406250108392300, 5.444914386472304635 ) ) ;
#6328=CARTESIAN_POINT ( 'NONE',  ( -13.14518615778179722, 39.90859375108393436, -5.444914386472297529 ) ) ;
#6336=CARTESIAN_POINT ( 'NONE',  ( 2.493653234604083739E-15, 36.43593749999999432, 13.57481594606304576 ) ) ;
#6337=CARTESIAN_POINT ( 'NONE',  ( 5.444914386472297529, 36.33671875108394289, -13.14518615778179900 ) ) ;
#6344=EDGE_CURVE ( 'NONE', #7430, #8989, #9961, .T. ) ;
#6345=CARTESIAN_POINT ( 'NONE',  ( -9.598844408820458085, 38.61875000216787157, -9.598844408820458085 ) ) ;
#6347=EDGE_CURVE ( 'NONE', #17326, #14317, #1265, .T. ) ;
#6348=( BOUNDED_CURVE ( )  B_SPLINE_CURVE ( 2, ( #19304, #8607, #6196, #10307, #3644, #12725, #12307, #2063, #27727, #8188, #1513, #8467, #1928, #10596, #25577, #28003, #28140, #6328, #15003, #10167, #27586, #6061, #8046, #16743, #25442, #2208, #24145, #17438, #6745, #4338, #17579, #636, #12994, #6603, #15720, #25997, #65, #2632, #20156, #11146, #24423, #26285, #21734, #11436, #7024, #2772, #2351, #9036, #15287, #2486, #17728, #26137, #6890, #9310, #26431, #11007, #4622, #23860, #15576, #6468, #8747, #19862, #11292, #15430, #20014, #13279, #4482, #24283, #22009, #15142, #349, #19719, #13573, #24005, #17869, #10871, #13138, #4911, #22296, #4764, #19582, #21875, #204, #8889, #13425, #26573, #22151, #9176, #495, #14000, #12000, #18444, #1209, #26717, #24995, #5334, #5616, #20725, #16292, #7743, #22863, #16431, #1067, #18150, #22580, #3190, #5474, #2905, #7311, #13716, #9875, #3330, #7452, #16146, #5191, #1344, #779, #9451, #20442, #18581, #14282, #13855, #3049, #9594, #14144, #15860, #5050, #27285, #20862, #24854, #25129, #22724, #18297, #26864, #27005, #23000, #3470, #15998, #27151, #7603, #11861, #12137, #11717, #18007, #7164, #20583, #9736, #24714, #924, #24569, #22437, #11574, #20294, #8161, #10425, #3616, #25265, #17123, #6031, #10568, #18850, #16573, #21561, #25552, #19277, #25826, #27558, #16853, #1621, #3889, #8016, #12834, #18719, #14977, #6300, #23696, #3754, #18988, #14695, #12275, #7880, #21277, #10008 ),
 .UNSPECIFIED., .F., .F. ) 
 B_SPLINE_CURVE_WITH_KNOTS ( ( 3, 2, 2, 2, 2, 2, 2, 2, 2, 2, 2, 2, 2, 2, 2, 2, 2, 2, 2, 2, 2, 2, 2, 2, 2, 2, 2, 2, 2, 2, 2, 2, 2, 2, 2, 2, 2, 2, 2, 2, 2, 2, 2, 2, 2, 2, 2, 2, 2, 2, 2, 2, 2, 2, 2, 2, 2, 2, 2, 2, 2, 2, 2, 2, 2, 2, 2, 2, 2, 2, 2, 2, 2, 2, 2, 2, 2, 2, 2, 2, 2, 2, 2, 2, 2, 2, 2, 2, 2, 2, 2, 3 ),
 ( 0.000000000000000000, 0.01041666666666666609, 0.02083333333333333218, 0.03125000000000000000, 0.04166666666666666435, 0.05208333333333333565, 0.06250000000000000000, 0.07291666666666667129, 0.08333333333333332871, 0.09375000000000000000, 0.1041666666666666713, 0.1145833333333333287, 0.1250000000000000000, 0.1354166666666666574, 0.1458333333333333426, 0.1562499999999999722, 0.1666666666666666574, 0.1770833333333333426, 0.1875000000000000000, 0.1979166666666666574, 0.2083333333333333426, 0.2187500000000000278, 0.2291666666666666574, 0.2395833333333333426, 0.2500000000000000000, 0.2604166666666666852, 0.2708333333333333148, 0.2812500000000000000, 0.2916666666666666852, 0.3020833333333333148, 0.3124999999999999445, 0.3229166666666666852, 0.3333333333333333148, 0.3437500000000000000, 0.3541666666666666852, 0.3645833333333333148, 0.3750000000000000000, 0.3854166666666666852, 0.3958333333333333148, 0.4062500000000000000, 0.4166666666666666852, 0.4270833333333333148, 0.4375000000000000555, 0.4479166666666666852, 0.4583333333333333148, 0.4687500000000000000, 0.4791666666666666852, 0.4895833333333333148, 0.5000000000000000000, 0.5104166666666666297, 0.5208333333333333703, 0.5312500000000000000, 0.5416666666666666297, 0.5520833333333333703, 0.5625000000000000000, 0.5729166666666666297, 0.5833333333333333703, 0.5937500000000000000, 0.6041666666666666297, 0.6145833333333333703, 0.6249999999999998890, 0.6354166666666666297, 0.6458333333333333703, 0.6562500000000000000, 0.6666666666666666297, 0.6770833333333333703, 0.6875000000000000000, 0.6979166666666666297, 0.7083333333333333703, 0.7187500000000000000, 0.7291666666666666297, 0.7395833333333333703, 0.7500000000000000000, 0.7604166666666666297, 0.7708333333333333703, 0.7812500000000000000, 0.7916666666666666297, 0.8020833333333333703, 0.8125000000000000000, 0.8229166666666666297, 0.8333333333333333703, 0.8437500000000000000, 0.8541666666666666297, 0.8645833333333333703, 0.8750000000000001110, 0.8854166666666666297, 0.8958333333333333703, 0.9062500000000000000, 0.9166666666666666297, 0.9270833333333333703, 0.9375000000000000000, 0.9448587001587775980 ),
 .UNSPECIFIED. ) 
 CURVE ( )  GEOMETRIC_REPRESENTATION_ITEM ( )  RATIONAL_B_SPLINE_CURVE ( ( 1.000000000000000000, 0.9238795325112867385, 1.000000000000000000, 0.9238795325112867385, 1.000000000000000000, 0.9238795325112867385, 1.000000000000000000, 0.9238795325112867385, 1.000000000000000000, 0.9238795325112867385, 1.000000000000000000, 0.9238795325112867385, 1.000000000000000000, 0.9238795325112867385, 1.000000000000000000, 0.9238795325112867385, 1.000000000000000000, 0.9238795325112867385, 1.000000000000000000, 0.9238795325112867385, 1.000000000000000000, 0.9238795325112867385, 1.000000000000000000, 0.9238795325112867385, 1.000000000000000000, 0.9238795325112867385, 1.000000000000000000, 0.9238795325112867385, 1.000000000000000000, 0.9238795325112867385, 1.000000000000000000, 0.9238795325112867385, 1.000000000000000000, 0.9238795325112867385, 1.000000000000000000, 0.9238795325112867385, 1.000000000000000000, 0.9238795325112867385, 1.000000000000000000, 0.9238795325112867385, 1.000000000000000000, 0.9238795325112867385, 1.000000000000000000, 0.9238795325112867385, 1.000000000000000000, 0.9238795325112867385, 1.000000000000000000, 0.9238795325112867385, 1.000000000000000000, 0.9238795325112867385, 1.000000000000000000, 0.9238795325112867385, 1.000000000000000000, 0.9238795325112867385, 1.000000000000000000, 0.9238795325112867385, 1.000000000000000000, 0.9238795325112867385, 1.000000000000000000, 0.9238795325112867385, 1.000000000000000000, 0.9238795325112867385, 1.000000000000000000, 0.9238795325112867385, 1.000000000000000000, 0.9238795325112867385, 1.000000000000000000, 0.9238795325112867385, 1.000000000000000000, 0.9238795325112867385, 1.000000000000000000, 0.9238795325112867385, 1.000000000000000000, 0.9238795325112867385, 1.000000000000000000, 0.9238795325112867385, 1.000000000000000000, 0.9238795325112867385, 1.000000000000000000, 0.9238795325112867385, 1.000000000000000000, 0.9238795325112867385, 1.000000000000000000, 0.9238795325112867385, 1.000000000000000000, 0.9238795325112867385, 1.000000000000000000, 0.9238795325112867385, 1.000000000000000000, 0.9238795325112867385, 1.000000000000000000, 0.9238795325112867385, 1.000000000000000000, 0.9238795325112867385, 1.000000000000000000, 0.9238795325112867385, 1.000000000000000000, 0.9238795325112867385, 1.000000000000000000, 0.9238795325112867385, 1.000000000000000000, 0.9238795325112867385, 1.000000000000000000, 0.9238795325112867385, 1.000000000000000000, 0.9238795325112867385, 1.000000000000000000, 0.9238795325112867385, 1.000000000000000000, 0.9238795325112867385, 1.000000000000000000, 0.9238795325112867385, 1.000000000000000000, 0.9238795325112867385, 1.000000000000000000, 0.9238795325112867385, 1.000000000000000000, 0.9238795325112867385, 1.000000000000000000, 0.9238795325112867385, 1.000000000000000000, 0.9238795325112867385, 1.000000000000000000, 0.9238795325112867385, 1.000000000000000000, 0.9238795325112867385, 1.000000000000000000, 0.9238795325112867385, 1.000000000000000000, 0.9238795325112867385, 1.000000000000000000, 0.9238795325112867385, 1.000000000000000000, 0.9238795325112867385, 1.000000000000000000, 0.9238795325112867385, 1.000000000000000000, 0.9238795325112867385, 1.000000000000000000, 0.9238795325112867385, 1.000000000000000000, 0.9238795325112867385, 1.000000000000000000, 0.9238795325112867385, 1.000000000000000000, 0.9238795325112867385, 1.000000000000000000, 0.9238795325112867385, 1.000000000000000000, 0.9238795325112867385, 1.000000000000000000, 0.9238795325112867385, 1.000000000000000000, 0.9238795325112867385, 1.000000000000000000, 0.9238795325112867385, 1.000000000000000000, 0.9238795325112867385, 1.000000000000000000, 0.9238795325112867385, 1.000000000000000000, 0.9238795325112867385, 1.000000000000000000, 0.9238795325112867385, 1.000000000000000000, 0.9238795325112867385, 1.000000000000000000, 0.9238795325112867385, 1.000000000000000000, 0.9238795325112867385, 1.000000000000000000, 0.9238795325112867385, 1.000000000000000000, 0.9238795325112867385, 1.000000000000000000, 0.9238795325112867385, 1.000000000000000000, 0.9238795325112867385, 1.000000000000000000, 0.9238795325112867385, 1.000000000000000000, 0.9462258211652395667, 0.9684275895297407288 ) ) 
 REPRESENTATION_ITEM ( '' )  );
#6369=DIRECTION ( 'NONE',  ( 0.000000000000000000, 0.000000000000000000, -1.000000000000000000 ) ) ;
#6370=CARTESIAN_POINT ( 'NONE',  ( 1.907364849565526780E-15, 40.99999999999999289, 15.57481594606304576 ) ) ;
#6380=AXIS2_PLACEMENT_3D ( 'NONE', #11253, #19970, #6986 ) ;
#6384=CARTESIAN_POINT ( 'NONE',  ( -8.312177448680279460E-16, 35.24531249999999716, -13.57481594606304576 ) ) ;
#6385=( GEOMETRIC_REPRESENTATION_CONTEXT ( 3 ) GLOBAL_UNCERTAINTY_ASSIGNED_CONTEXT ( ( #23810 ) ) GLOBAL_UNIT_ASSIGNED_CONTEXT ( ( #15640, #15061, #19778 ) ) REPRESENTATION_CONTEXT ( 'NONE', 'WORKASPACE' ) );
#6390=EDGE_CURVE ( 'NONE', #18296, #24795, #20720, .T. ) ;
#6397=CARTESIAN_POINT ( 'NONE',  ( 9.295050272127047819, 38.46992187608393010, 9.295050272127046043 ) ) ;
#6409=ORIENTED_EDGE ( 'NONE', *, *, #22053, .T. ) ;
#6423=CARTESIAN_POINT ( 'NONE',  ( -13.14518615778179544, 35.79101562608393294, 0.000000000000000000 ) ) ;
#6446=ORIENTED_EDGE ( 'NONE', *, *, #20656, .F. ) ;
#6461=CARTESIAN_POINT ( 'NONE',  ( 13.14518615778179900, 38.02343750108395426, -5.444914386472297529 ) ) ;
#6468=CARTESIAN_POINT ( 'NONE',  ( 5.444914386472302859, 37.82500000108392868, 13.14518615778179189 ) ) ;
#6474=CARTESIAN_POINT ( 'NONE',  ( 2.493653234604083739E-15, 35.64218749999999147, 13.57481594606304576 ) ) ;
#6475=CARTESIAN_POINT ( 'NONE',  ( -13.14518615778179900, 36.53515625108392584, -5.444914386472297529 ) ) ;
#6491=CARTESIAN_POINT ( 'NONE',  ( -9.598844408820454532, 37.13046874999999147, 9.598844408820459861 ) ) ;
#6509=CARTESIAN_POINT ( 'NONE',  ( 0.000000000000000000, 40.99999999999999289, 0.000000000000000000 ) ) ;
#6511=CARTESIAN_POINT ( 'NONE',  ( -9.295050272127046043, 35.89023437608393152, -9.295050272127046043 ) ) ;
#6512=CARTESIAN_POINT ( 'NONE',  ( -8.312177448680279460E-16, 37.72578125216787726, -13.57481594606304576 ) ) ;
#6528=CARTESIAN_POINT ( 'NONE',  ( -5.444914386472297529, 39.61093750108393152, -13.14518615778179900 ) ) ;
#6532=CARTESIAN_POINT ( 'NONE',  ( -8.312177448680279460E-16, 32.86406249999999574, -13.57481594606304576 ) ) ;
#6555=CARTESIAN_POINT ( 'NONE',  ( -5.444914386472299306, 35.14609375108393152, 13.14518615778179722 ) ) ;
#6556=DIRECTION ( 'NONE',  ( 0.000000000000000000, 0.000000000000000000, -1.000000000000000000 ) ) ;
#6598=CARTESIAN_POINT ( 'NONE',  ( 9.295050272127047819, 37.87460937608393863, 9.295050272127046043 ) ) ;
#6603=CARTESIAN_POINT ( 'NONE',  ( -13.14518615778179722, 39.11484375108393863, -5.444914386472297529 ) ) ;
#6609=CARTESIAN_POINT ( 'NONE',  ( -13.57481594606304576, 37.87460937499999147, 5.622872871577880183 ) ) ;
#6610=CARTESIAN_POINT ( 'NONE',  ( 5.444914386472297529, 37.13046875108393152, -13.14518615778179900 ) ) ;
#6628=CARTESIAN_POINT ( 'NONE',  ( -9.598844408820458085, 36.93203124999999432, -9.598844408820458085 ) ) ;
#6646=CARTESIAN_POINT ( 'NONE',  ( 13.14518615778179900, 38.02343750108395426, -5.444914386472297529 ) ) ;
#6647=CARTESIAN_POINT ( 'NONE',  ( 13.57481594606304931, 38.27148437716787299, 5.622872871577869525 ) ) ;
#6657=CARTESIAN_POINT ( 'NONE',  ( 2.493653234604083739E-15, 34.15390625216787157, 13.57481594606304576 ) ) ;
#6666=CARTESIAN_POINT ( 'NONE',  ( -9.295050272127044266, 35.89023437608393152, 9.295050272127047819 ) ) ;
#6692=CARTESIAN_POINT ( 'NONE',  ( -5.444914386472297529, 34.84843750108393579, -13.14518615778179722 ) ) ;
#6705=DIRECTION ( 'NONE',  ( -0.000000000000000000, -1.000000000000000000, -0.000000000000000000 ) ) ;
#6734=CARTESIAN_POINT ( 'NONE',  ( 13.57481594606304931, 37.37851562499999858, 5.622872871577868636 ) ) ;
#6739=CARTESIAN_POINT ( 'NONE',  ( 9.295050272127047819, 39.46210937608393721, 9.295050272127046043 ) ) ;
#6745=CARTESIAN_POINT ( 'NONE',  ( 2.414731522848535132E-15, 39.36289062608393152, 13.14518615778179544 ) ) ;
#6746=CARTESIAN_POINT ( 'NONE',  ( -9.598844408820454532, 39.61093750216787868, 9.598844408820459861 ) ) ;
#6747=CARTESIAN_POINT ( 'NONE',  ( -8.312177448680279460E-16, 36.93203125216787441, -13.57481594606304576 ) ) ;
#6753=CARTESIAN_POINT ( 'NONE',  ( -13.57481594606304576, 36.28710937499999289, 5.622872871577880183 ) ) ;
#6754=CARTESIAN_POINT ( 'NONE',  ( 13.14518615778179900, 38.61875000108393152, -5.444914386472297529 ) ) ;
#6760=( BOUNDED_CURVE ( )  B_SPLINE_CURVE ( 2, ( #18456, #7614, #25007, #16441, #14434, #7890, #3341, #12425, #21143 ),
 .UNSPECIFIED., .F., .F. ) 
 B_SPLINE_CURVE_WITH_KNOTS ( ( 3, 2, 2, 2, 3 ),
 ( 0.7708333333333333703, 0.7812500000000000000, 0.7916666666666665186, 0.8020833333333332593, 0.8124999999999998890 ),
 .UNSPECIFIED. ) 
 CURVE ( )  GEOMETRIC_REPRESENTATION_ITEM ( )  RATIONAL_B_SPLINE_CURVE ( ( 1.000000000000000000, 0.9238795325112867385, 1.000000000000000000, 0.9238795325112867385, 1.000000000000000000, 0.9238795325112867385, 1.000000000000000000, 0.9238795325112875156, 0.9999999999999992228 ) ) 
 REPRESENTATION_ITEM ( '' )  );
#6771=STYLED_ITEM ( 'NONE', ( #3077 ), #15807 ) ;
#6783=CARTESIAN_POINT ( 'NONE',  ( 2.493653234604083739E-15, 39.61093749999999147, 13.57481594606304576 ) ) ;
#6788=LINE ( 'NONE', #19486, #19093 ) ;
#6789=CARTESIAN_POINT ( 'NONE',  ( 13.14518615778179544, 36.38632812608393863, -1.609821015232357215E-15 ) ) ;
#6790=CARTESIAN_POINT ( 'NONE',  ( 13.57481594606304753, 35.98945312716787015, -5.622872871577873077 ) ) ;
#6810=CARTESIAN_POINT ( 'NONE',  ( 13.14518615778179900, 36.13828125108393863, 5.444914386472293977 ) ) ;
#6813=CARTESIAN_POINT ( 'NONE',  ( 0.000000000000000000, 40.99999999999999289, 0.000000000000000000 ) ) ;
#6817=ORIENTED_EDGE ( 'NONE', *, *, #26815, .F. ) ;
#6837=CARTESIAN_POINT ( 'NONE',  ( 13.14518615778179544, 35.39414062608393152, -1.609821015232357215E-15 ) ) ;
#6859=DIRECTION ( 'NONE',  ( -0.000000000000000000, -1.000000000000000000, -0.000000000000000000 ) ) ;
#6883=CARTESIAN_POINT ( 'NONE',  ( 13.14518615778179544, 40.35507812608393863, -1.609821015232357215E-15 ) ) ;
#6885=( BOUNDED_CURVE ( )  B_SPLINE_CURVE ( 2, ( #68, #12728, #13140, #23862, #25999, #2065, #23727, #11149, #26139 ),
 .UNSPECIFIED., .F., .F. ) 
 B_SPLINE_CURVE_WITH_KNOTS ( ( 3, 2, 2, 2, 3 ),
 ( 0.3125000000000002220, 0.3229166666666668517, 0.3333333333333334259, 0.3437500000000000555, 0.3541666666666666852 ),
 .UNSPECIFIED. ) 
 CURVE ( )  GEOMETRIC_REPRESENTATION_ITEM ( )  RATIONAL_B_SPLINE_CURVE ( ( 0.9999999999999983347, 0.9238795325112884038, 1.000000000000000000, 0.9238795325112867385, 1.000000000000000000, 0.9238795325112867385, 1.000000000000000000, 0.9238795325112867385, 1.000000000000000000 ) ) 
 REPRESENTATION_ITEM ( '' )  );
#6890=CARTESIAN_POINT ( 'NONE',  ( -8.049105076161786076E-16, 38.17226562608394147, -13.14518615778179544 ) ) ;
#6895=CARTESIAN_POINT ( 'NONE',  ( -5.622872871577873077, 35.59257812499999574, 13.57481594606304753 ) ) ;
#6896=CARTESIAN_POINT ( 'NONE',  ( -9.295050272127044266, 37.47773437608393010, 9.295050272127047819 ) ) ;
#6915=CARTESIAN_POINT ( 'NONE',  ( 1.662435489736055892E-15, 40.99999999999999289, 13.57481594606304576 ) ) ;
#6923=CARTESIAN_POINT ( 'NONE',  ( 5.622872871577924592, 33.31054687499999289, 13.57481594606299957 ) ) ;
#6930=( BOUNDED_CURVE ( )  B_SPLINE_CURVE ( 2, ( #4787, #17889, #26596, #7042, #24445, #24733, #13594, #5213, #2790 ),
 .UNSPECIFIED., .F., .F. ) 
 B_SPLINE_CURVE_WITH_KNOTS ( ( 3, 2, 2, 2, 3 ),
 ( 0.4375000000000003331, 0.4479166666666669627, 0.4583333333333335369, 0.4687500000000001665, 0.4791666666666667962 ),
 .UNSPECIFIED. ) 
 CURVE ( )  GEOMETRIC_REPRESENTATION_ITEM ( )  RATIONAL_B_SPLINE_CURVE ( ( 0.9999999999999975575, 0.9238795325112891810, 1.000000000000000000, 0.9238795325112867385, 1.000000000000000000, 0.9238795325112867385, 1.000000000000000000, 0.9238795325112859613, 1.000000000000000888 ) ) 
 REPRESENTATION_ITEM ( '' )  );
#6931=CARTESIAN_POINT ( 'NONE',  ( 5.444914386472297529, 37.32890625108393579, -13.14518615778179900 ) ) ;
#6932=CARTESIAN_POINT ( 'NONE',  ( 5.622872871577878406, 36.58476562716787583, 13.57481594606304576 ) ) ;
#6942=FACE_OUTER_BOUND ( 'NONE', #26574, .T. ) ;
#6950=DIRECTION ( 'NONE',  ( 0.000000000000000000, 0.000000000000000000, -1.000000000000000000 ) ) ;
#6952=CARTESIAN_POINT ( 'NONE',  ( -5.444914386472299306, 36.73359375108393010, 13.14518615778179722 ) ) ;
#6968=CARTESIAN_POINT ( 'NONE',  ( 5.622872871577780707, 34.40195312499999858, -13.57481594606313990 ) ) ;
#6978=CARTESIAN_POINT ( 'NONE',  ( 5.444914386472297529, 33.16171875108393152, -13.14518615778179722 ) ) ;
#6986=DIRECTION ( 'NONE',  ( 0.000000000000000000, 0.000000000000000000, -1.000000000000000000 ) ) ;
#7016=EDGE_CURVE ( 'NONE', #20608, #19588, #17692, .T. ) ;
#7019=CARTESIAN_POINT ( 'NONE',  ( 2.414731522848535132E-15, 35.39414062608393863, 13.14518615778179544 ) ) ;
#7023=CARTESIAN_POINT ( 'NONE',  ( 0.000000000000000000, 30.99999999999999645, -15.57481594606304576 ) ) ;
#7024=CARTESIAN_POINT ( 'NONE',  ( 2.414731522848535132E-15, 38.56914062608393579, 13.14518615778179544 ) ) ;
#7029=CARTESIAN_POINT ( 'NONE',  ( -13.57481594606304576, 33.06249999999999289, 0.000000000000000000 ) ) ;
#7030=CARTESIAN_POINT ( 'NONE',  ( 2.414731522848535132E-15, 33.60820312608392868, 13.14518615778179544 ) ) ;
#7033=CARTESIAN_POINT ( 'NONE',  ( 2.493653234604083739E-15, 35.74140625216787015, 13.57481594606304576 ) ) ;
#7042=CARTESIAN_POINT ( 'NONE',  ( 13.57481594606304753, 36.68398437500000142, -5.622872871577873966 ) ) ;
#7067=CARTESIAN_POINT ( 'NONE',  ( -13.57481594606304576, 40.30546875216787583, 0.000000000000000000 ) ) ;
#7068=CARTESIAN_POINT ( 'NONE',  ( -13.14518615778179189, 33.65781250108393152, 5.444914386472304635 ) ) ;
#7069=CARTESIAN_POINT ( 'NONE',  ( -9.598844408820454532, 34.84843750216787583, 9.598844408820459861 ) ) ;
#7088=CARTESIAN_POINT ( 'NONE',  ( -8.049105076161786076E-16, 34.79882812608393294, -13.14518615778179544 ) ) ;
#7117=CARTESIAN_POINT ( 'NONE',  ( 3.755638265659908104, 31.58960998161716560, -13.14518615778179722 ) ) ;
#7159=CARTESIAN_POINT ( 'NONE',  ( 2.414731522848535132E-15, 36.18789062608393436, 13.14518615778179544 ) ) ;
#7164=CARTESIAN_POINT ( 'NONE',  ( -13.14518615778179544, 33.60820312608393579, 0.000000000000000000 ) ) ;
#7169=CARTESIAN_POINT ( 'NONE',  ( 9.598844408820459861, 34.15390624999999858, 9.598844408820456309 ) ) ;
#7170=CARTESIAN_POINT ( 'NONE',  ( 13.14518615778179900, 34.55078125108393294, 5.444914386472293977 ) ) ;
#7203=CARTESIAN_POINT ( 'NONE',  ( 5.444914386472297529, 34.15390625108393863, -13.14518615778179900 ) ) ;
#7204=CARTESIAN_POINT ( 'NONE',  ( 9.598844408820459861, 33.45937500216787441, 9.598844408820456309 ) ) ;
#7230=CARTESIAN_POINT ( 'NONE',  ( 9.295050272127046043, 37.08085937608393579, -9.295050272127046043 ) ) ;
#7244=LINE ( 'NONE', #13934, #13625 ) ;
#7249=VECTOR ( 'NONE', #2316, 1000.000000000000000 ) ;
#7261=CARTESIAN_POINT ( 'NONE',  ( 6.944423797152706079, 31.55306878032414986, -11.16113333171310451 ) ) ;
#7262=CARTESIAN_POINT ( 'NONE',  ( 9.598844408820459861, 36.63437500216787157, 9.598844408820456309 ) ) ;
#7290=ORIENTED_EDGE ( 'NONE', *, *, #10285, .T. ) ;
#7305=CARTESIAN_POINT ( 'NONE',  ( 13.14518615778179900, 34.84843750108393579, -5.444914386472297529 ) ) ;
#7311=CARTESIAN_POINT ( 'NONE',  ( 2.414731522848535132E-15, 35.39414062608393863, 13.14518615778179544 ) ) ;
#7317=CARTESIAN_POINT ( 'NONE',  ( -8.312177448680279460E-16, 33.65781249999999147, -13.57481594606304576 ) ) ;
#7318=CARTESIAN_POINT ( 'NONE',  ( -8.049105076161786076E-16, 34.00507812608393721, -13.14518615778179544 ) ) ;
#7331=CARTESIAN_POINT ( 'NONE',  ( -5.622872871577737186, 34.89804687716787157, 13.57481594606318254 ) ) ;
#7351=CARTESIAN_POINT ( 'NONE',  ( 13.14518615778179544, 34.00507812608393721, -1.609821015232357215E-15 ) ) ;
#7352=CARTESIAN_POINT ( 'NONE',  ( -9.598844408820454532, 33.26093750216787726, 9.598844408820459861 ) ) ;
#7363=CARTESIAN_POINT ( 'NONE',  ( -13.57481594606304753, 31.52460937716787370, -5.622872871577872189 ) ) ;
#7372=CARTESIAN_POINT ( 'NONE',  ( 5.444914386472297529, 33.95546875108393436, -13.14518615778179900 ) ) ;
#7402=CARTESIAN_POINT ( 'NONE',  ( 13.14518615778179722, 34.65000000108393152, -5.444914386472297529 ) ) ;
#7423=CARTESIAN_POINT ( 'NONE',  ( -13.36000105192242060, 40.87597656304196647, 0.000000000000000000 ) ) ;
#7424=DIRECTION ( 'NONE',  ( 0.000000000000000000, 0.000000000000000000, -1.000000000000000000 ) ) ;
#7430=VERTEX_POINT ( 'NONE', #22893 ) ;
#7445=CARTESIAN_POINT ( 'NONE',  ( -13.14518615778179189, 34.45156250108394147, 5.444914386472304635 ) ) ;
#7452=CARTESIAN_POINT ( 'NONE',  ( -13.14518615778179544, 35.19570312608393436, 0.000000000000000000 ) ) ;
#7458=CARTESIAN_POINT ( 'NONE',  ( -13.57481594606304576, 32.31835937499999289, 5.622872871577880183 ) ) ;
#7459=CARTESIAN_POINT ( 'NONE',  ( -8.049105076161786076E-16, 34.79882812608393294, -13.14518615778179544 ) ) ;
#7465=ORIENTED_EDGE ( 'NONE', *, *, #3251, .T. ) ;
#7494=CARTESIAN_POINT ( 'NONE',  ( 9.295050272127047819, 33.11210937608393579, 9.295050272127046043 ) ) ;
#7495=CARTESIAN_POINT ( 'NONE',  ( 13.57481594606304576, 32.76484375216787015, -1.662435489736055892E-15 ) ) ;
#7518=CARTESIAN_POINT ( 'NONE',  ( 2.493653234604083739E-15, 40.40468749999999432, 13.57481594606304576 ) ) ;
#7520=CARTESIAN_POINT ( 'NONE',  ( 13.14518615778179900, 32.26875000108393721, -5.444914386472297529 ) ) ;
#7523=CARTESIAN_POINT ( 'NONE',  ( -13.57481594606304576, 37.92421875216787441, 0.000000000000000000 ) ) ;
#7541=DIRECTION ( 'NONE',  ( 0.000000000000000000, 0.000000000000000000, -1.000000000000000000 ) ) ;
#7546=ADVANCED_FACE ( 'NONE', ( #12580 ), #14726, .F. ) ;
#7550=CARTESIAN_POINT ( 'NONE',  ( -9.295050272127044266, 31.92148437608393508, 9.295050272127047819 ) ) ;
#7558=CARTESIAN_POINT ( 'NONE',  ( 2.493653234604083739E-15, 35.74140625216787015, 13.57481594606304576 ) ) ;
#7591=EDGE_CURVE ( 'NONE', #10432, #15088, #6348, .T. ) ;
#7594=CARTESIAN_POINT ( 'NONE',  ( 9.598844408820456309, 38.42031250216787441, -9.598844408820458085 ) ) ;
#7595=CARTESIAN_POINT ( 'NONE',  ( -5.444914386472299306, 36.13828125108393863, 13.14518615778179722 ) ) ;
#7603=CARTESIAN_POINT ( 'NONE',  ( 5.444914386472302859, 33.85625000108393579, 13.14518615778179189 ) ) ;
#7606=DIRECTION ( 'NONE',  ( 0.000000000000000000, 1.000000000000000000, 0.000000000000000000 ) ) ;
#7609=CARTESIAN_POINT ( 'NONE',  ( 9.598844408820456309, 33.55859375000000000, -9.598844408820458085 ) ) ;
#7610=CARTESIAN_POINT ( 'NONE',  ( 5.444914386472297529, 33.95546875108393436, -13.14518615778179900 ) ) ;
#7614=CARTESIAN_POINT ( 'NONE',  ( 5.622872871577870413, 32.91367187716787157, -13.57481594606304753 ) ) ;
#7616=ORIENTED_EDGE ( 'NONE', *, *, #25654, .T. ) ;
#7643=CARTESIAN_POINT ( 'NONE',  ( 9.295050272127046043, 32.51679687608393721, -9.295050272127046043 ) ) ;
#7644=CARTESIAN_POINT ( 'NONE',  ( 5.622872871577871301, 34.50117187716788436, -13.57481594606304753 ) ) ;
#7667=CARTESIAN_POINT ( 'NONE',  ( -9.295050272127046043, 31.72304687608393081, -9.295050272127046043 ) ) ;
#7726=CARTESIAN_POINT ( 'NONE',  ( -8.049105076161786076E-16, 37.97382812608393721, -13.14518615778179544 ) ) ;
#7735=CARTESIAN_POINT ( 'NONE',  ( -8.049105076161786076E-16, 34.20351562608394147, -13.14518615778179544 ) ) ;
#7740=CARTESIAN_POINT ( 'NONE',  ( 13.57481594606304931, 39.06523437716786873, 5.622872871577868636 ) ) ;
#7743=CARTESIAN_POINT ( 'NONE',  ( -5.444914386472297529, 35.84062500108394289, -13.14518615778179722 ) ) ;
#7750=CARTESIAN_POINT ( 'NONE',  ( -5.444914386472299306, 31.97109375108393436, 13.14518615778179722 ) ) ;
#7754=DIRECTION ( 'NONE',  ( -0.000000000000000000, -1.000000000000000000, -0.000000000000000000 ) ) ;
#7772=PLANE ( 'NONE',  #9709 ) ;
#7776=COLOUR_RGB ( '', 0.72549020, 0.75294118, 0.79215686) ;
#7785=CARTESIAN_POINT ( 'NONE',  ( -13.57481594606304576, 38.66835937499999432, 5.622872871577880183 ) ) ;
#7786=CARTESIAN_POINT ( 'NONE',  ( 9.598844408820456309, 32.07031250216787299, -9.598844408820458085 ) ) ;
#7809=CARTESIAN_POINT ( 'NONE',  ( 3.755639919285892248, 31.58960996655074993, -13.14518615778179544 ) ) ;
#7819=CARTESIAN_POINT ( 'NONE',  ( 9.598844408820456309, 33.55859375000000000, -9.598844408820458085 ) ) ;
#7862=ORIENTED_EDGE ( 'NONE', *, *, #18231, .T. ) ;
#7866=CARTESIAN_POINT ( 'NONE',  ( -9.295050272127046043, 38.86679687608393863, -9.295050272127046043 ) ) ;
#7878=CARTESIAN_POINT ( 'NONE',  ( 2.493653234604083739E-15, 38.91640625216786731, 13.57481594606304576 ) ) ;
#7880=CARTESIAN_POINT ( 'NONE',  ( -8.049105076161786076E-16, 31.82226562608393650, -13.14518615778179544 ) ) ;
#7886=CARTESIAN_POINT ( 'NONE',  ( 5.444914386472297529, 32.36796875108393579, -13.14518615778179900 ) ) ;
#7890=CARTESIAN_POINT ( 'NONE',  ( 13.57481594606304931, 32.71523437716787441, 5.622872871577868636 ) ) ;
#7892=CARTESIAN_POINT ( 'NONE',  ( -8.312177448680279460E-16, 35.24531249999999716, -13.57481594606304576 ) ) ;
#7917=CARTESIAN_POINT ( 'NONE',  ( 2.493653234604083739E-15, 37.32890625216786873, 13.57481594606304576 ) ) ;
#7918=CARTESIAN_POINT ( 'NONE',  ( -9.295050272127046043, 31.92148437608393508, -9.295050272127046043 ) ) ;
#7919=CARTESIAN_POINT ( 'NONE',  ( 7.171391395016640580, 31.30502190640808990, -11.52591746582321974 ) ) ;
#7927=DIRECTION ( 'NONE',  ( 0.000000000000000000, 0.000000000000000000, -1.000000000000000000 ) ) ;
#7941=CARTESIAN_POINT ( 'NONE',  ( 0.000000000000000000, 30.99999999999999645, -13.57481594606304576 ) ) ;
#7953=VERTEX_POINT ( 'NONE', #22406 ) ;
#7956=CARTESIAN_POINT ( 'NONE',  ( 13.57481594606304753, 39.16445312716788152, -5.622872871577873077 ) ) ;
#7999=CARTESIAN_POINT ( 'NONE',  ( -9.295050272127044266, 38.27148437608393294, 9.295050272127047819 ) ) ;
#8015=VERTEX_POINT ( 'NONE', #18120 ) ;
#8016=CARTESIAN_POINT ( 'NONE',  ( 9.295050272127047819, 32.31835937608393294, 9.295050272127046043 ) ) ;
#8018=( BOUNDED_CURVE ( )  B_SPLINE_CURVE ( 2, ( #5073, #7331, #9195, #20034, #3211, #2924, #11879, #15741, #20603 ),
 .UNSPECIFIED., .F., .F. ) 
 B_SPLINE_CURVE_WITH_KNOTS ( ( 3, 2, 2, 2, 3 ),
 ( 0.5624999999999996669, 0.5729166666666664076, 0.5833333333333332593, 0.5937500000000001110, 0.6041666666666668517 ),
 .UNSPECIFIED. ) 
 CURVE ( )  GEOMETRIC_REPRESENTATION_ITEM ( )  RATIONAL_B_SPLINE_CURVE ( ( 1.000000000000002442, 0.9238795325112842960, 1.000000000000000000, 0.9238795325112867385, 1.000000000000000000, 0.9238795325112867385, 1.000000000000000000, 0.9238795325112850731, 1.000000000000001554 ) ) 
 REPRESENTATION_ITEM ( '' )  );
#8040=ORIENTED_EDGE ( 'NONE', *, *, #17718, .F. ) ;
#8044=FACE_BOUND ( 'NONE', #13380, .T. ) ;
#8046=CARTESIAN_POINT ( 'NONE',  ( 9.295050272127046043, 39.66054687608393436, -9.295050272127046043 ) ) ;
#8052=ORIENTED_EDGE ( 'NONE', *, *, #17839, .T. ) ;
#8054=CARTESIAN_POINT ( 'NONE',  ( -9.598844408820458085, 40.90078124999999432, -9.598844408820458085 ) ) ;
#8055=CARTESIAN_POINT ( 'NONE',  ( 9.295050272127047819, 39.26367187608393294, 9.295050272127046043 ) ) ;
#8078=AXIS2_PLACEMENT_3D ( 'NONE', #8488, #21184, #5940 ) ;
#8086=LINE ( 'NONE', #5263, #22319 ) ;
#8095=CARTESIAN_POINT ( 'NONE',  ( -5.444914386472297529, 39.01562500108394005, -13.14518615778179900 ) ) ;
#8096=CARTESIAN_POINT ( 'NONE',  ( 5.622872871577871301, 40.05742187716786873, -13.57481594606304753 ) ) ;
#8099=EDGE_CURVE ( 'NONE', #28027, #947, #7244, .T. ) ;
#8114=CARTESIAN_POINT ( 'NONE',  ( 13.14518615778179900, 39.41250000108393436, -5.444914386472297529 ) ) ;
#8118=CARTESIAN_POINT ( 'NONE',  ( 0.000000000000000000, 40.99999999999999289, -13.57481594606304576 ) ) ;
#8134=( BOUNDED_CURVE ( )  B_SPLINE_CURVE ( 2, ( #5164, #22550, #22697, #3019, #26978, #5306, #20559, #13969, #11835 ),
 .UNSPECIFIED., .F., .T. ) 
 B_SPLINE_CURVE_WITH_KNOTS ( ( 3, 2, 2, 2, 3 ),
 ( 0.02083333333333358892, 0.03125000000000020123, 0.04166666666666681007, 0.05208333333333342585, 0.06250000000000004163 ),
 .UNSPECIFIED. ) 
 CURVE ( )  GEOMETRIC_REPRESENTATION_ITEM ( )  RATIONAL_B_SPLINE_CURVE ( ( 0.9999999999999981126, 0.9238795325112886259, 1.000000000000000000, 0.9238795325112867385, 1.000000000000000000, 0.9238795325112867385, 1.000000000000000000, 0.9238795325112864054, 1.000000000000000222 ) ) 
 REPRESENTATION_ITEM ( '' )  );
#8142=CARTESIAN_POINT ( 'NONE',  ( -9.295050272127046043, 39.66054687608393436, -9.295050272127046043 ) ) ;
#8153=CARTESIAN_POINT ( 'NONE',  ( -9.295050272127046043, 33.50898437608393010, -9.295050272127046043 ) ) ;
#8161=CARTESIAN_POINT ( 'NONE',  ( 13.14518615778179722, 33.16171875108393863, 5.444914386472293977 ) ) ;
#8166=CARTESIAN_POINT ( 'NONE',  ( -13.57481594606304576, 32.26874999999999716, 0.000000000000000000 ) ) ;
#8175=CARTESIAN_POINT ( 'NONE',  ( -13.57481594606304576, 33.85624999999999574, 0.000000000000000000 ) ) ;
#8179=CARTESIAN_POINT ( 'NONE',  ( 5.622872871577786924, 31.82226562716788365, 13.57481594606313813 ) ) ;
#8188=CARTESIAN_POINT ( 'NONE',  ( 13.14518615778179722, 40.30546875108393579, 5.444914386472293977 ) ) ;
#8194=CARTESIAN_POINT ( 'NONE',  ( -9.598844408820454532, 39.51171874999999289, 9.598844408820459861 ) ) ;
#8195=CARTESIAN_POINT ( 'NONE',  ( -5.444914386472297529, 39.61093750108393152, -13.14518615778179900 ) ) ;
#8230=CARTESIAN_POINT ( 'NONE',  ( 13.14518615778179544, 38.76757812608393294, -1.609821015232357215E-15 ) ) ;
#8249=CARTESIAN_POINT ( 'NONE',  ( -9.295050272127044266, 39.06523437608392868, 9.295050272127047819 ) ) ;
#8252=CARTESIAN_POINT ( 'NONE',  ( 6.944423797152706079, 31.55306878032414986, -11.16113333171310451 ) ) ;
#8275=CARTESIAN_POINT ( 'NONE',  ( 5.444914386472297529, 39.51171875108393294, -13.14518615778179722 ) ) ;
#8291=EDGE_CURVE ( 'NONE', #8513, #11798, #6788, .T. ) ;
#8319=CARTESIAN_POINT ( 'NONE',  ( -9.295050272127046043, 32.51679687608393721, -9.295050272127046043 ) ) ;
#8325=DIRECTION ( 'NONE',  ( 0.000000000000000000, 0.000000000000000000, -1.000000000000000000 ) ) ;
#8331=ORIENTED_EDGE ( 'NONE', *, *, #24837, .F. ) ;
#8333=CARTESIAN_POINT ( 'NONE',  ( -9.598844408820458085, 39.31328124999999574, -9.598844408820458085 ) ) ;
#8334=CARTESIAN_POINT ( 'NONE',  ( -13.14518615778179189, 39.80937500108392868, 5.444914386472304635 ) ) ;
#8344=( BOUNDED_CURVE ( )  B_SPLINE_CURVE ( 2, ( #7917, #16612, #5793, #21037, #1906, #10572, #19281, #27979, #20760 ),
 .UNSPECIFIED., .F., .F. ) 
 B_SPLINE_CURVE_WITH_KNOTS ( ( 3, 2, 2, 2, 3 ),
 ( 0.3125000000000002220, 0.3229166666666668517, 0.3333333333333334259, 0.3437500000000000555, 0.3541666666666666852 ),
 .UNSPECIFIED. ) 
 CURVE ( )  GEOMETRIC_REPRESENTATION_ITEM ( )  RATIONAL_B_SPLINE_CURVE ( ( 0.9999999999999983347, 0.9238795325112884038, 1.000000000000000000, 0.9238795325112867385, 1.000000000000000000, 0.9238795325112867385, 1.000000000000000000, 0.9238795325112867385, 1.000000000000000000 ) ) 
 REPRESENTATION_ITEM ( '' )  );
#8363=ORIENTED_EDGE ( 'NONE', *, *, #17839, .F. ) ;
#8371=CARTESIAN_POINT ( 'NONE',  ( 2.414731522848535132E-15, 39.36289062608393152, 13.14518615778179544 ) ) ;
#8373=LINE ( 'NONE', #10218, #22520 ) ;
#8382=CARTESIAN_POINT ( 'NONE',  ( -13.57481594606304576, 38.61874999999999147, 0.000000000000000000 ) ) ;
#8387=CARTESIAN_POINT ( 'NONE',  ( -9.295050272127046043, 39.66054687608393436, -9.295050272127046043 ) ) ;
#8402=VERTEX_POINT ( 'NONE', #19762 ) ;
#8412=CARTESIAN_POINT ( 'NONE',  ( -13.14518615778179722, 36.53515625108393294, -5.444914386472297529 ) ) ;
#8449=CARTESIAN_POINT ( 'NONE',  ( 0.000000000000000000, 40.99999999999999289, 0.000000000000000000 ) ) ;
#8452=EDGE_CURVE ( 'NONE', #637, #21530, #23585, .T. ) ;
#8459=CARTESIAN_POINT ( 'NONE',  ( -9.295050272127044266, 40.05742187608393579, 9.295050272127047819 ) ) ;
#8467=CARTESIAN_POINT ( 'NONE',  ( 5.444914386472302859, 40.20625000108394431, 13.14518615778179189 ) ) ;
#8474=ADVANCED_FACE ( 'NONE', ( #19343 ), #8514, .F. ) ;
#8475=CARTESIAN_POINT ( 'NONE',  ( 5.622872871577878406, 35.69179687499999432, 13.57481594606304576 ) ) ;
#8476=CARTESIAN_POINT ( 'NONE',  ( -5.444914386472297529, 36.43593750108392726, -13.14518615778179900 ) ) ;
#8488=CARTESIAN_POINT ( 'NONE',  ( 0.000000000000000000, 40.99999999999999289, 0.000000000000000000 ) ) ;
#8513=VERTEX_POINT ( 'NONE', #2254 ) ;
#8514=CYLINDRICAL_SURFACE ( 'NONE', #2213, 13.57481594606304576 ) ;
#8515=CARTESIAN_POINT ( 'NONE',  ( 2.414731522848535132E-15, 40.15664062608393436, 13.14518615778179544 ) ) ;
#8527=CARTESIAN_POINT ( 'NONE',  ( 13.57481594606304753, 34.40195312716787157, -5.622872871577873966 ) ) ;
#8532=CARTESIAN_POINT ( 'NONE',  ( 9.295050272127046043, 37.87460937608393152, -9.295050272127046043 ) ) ;
#8550=( BOUNDED_CURVE ( )  B_SPLINE_CURVE ( 2, ( #22504, #24920, #25064, #24495, #995, #24643, #11644, #9525, #18225 ),
 .UNSPECIFIED., .F., .F. ) 
 B_SPLINE_CURVE_WITH_KNOTS ( ( 3, 2, 2, 2, 3 ),
 ( 0.5625000000000004441, 0.5729166666666669627, 0.5833333333333337034, 0.5937500000000002220, 0.6041666666666668517 ),
 .UNSPECIFIED. ) 
 CURVE ( )  GEOMETRIC_REPRESENTATION_ITEM ( )  RATIONAL_B_SPLINE_CURVE ( ( 0.9999999999999967804, 0.9238795325112899581, 1.000000000000000000, 0.9238795325112867385, 1.000000000000000000, 0.9238795325112867385, 1.000000000000000000, 0.9238795325112850731, 1.000000000000001554 ) ) 
 REPRESENTATION_ITEM ( '' )  );
#8553=ORIENTED_EDGE ( 'NONE', *, *, #23321, .T. ) ;
#8557=CARTESIAN_POINT ( 'NONE',  ( -9.295050272127046043, 37.27929687608393294, -9.295050272127046043 ) ) ;
#8602=CARTESIAN_POINT ( 'NONE',  ( 9.295050272127046043, 38.86679687608393863, -9.295050272127046043 ) ) ;
#8607=CARTESIAN_POINT ( 'NONE',  ( -13.14518615778179722, 40.70234375108392300, -5.444914386472297529 ) ) ;
#8613=EDGE_CURVE ( 'NONE', #17637, #13728, #5456, .T. ) ;
#8615=CARTESIAN_POINT ( 'NONE',  ( 9.598844408820459861, 37.32890624999999574, 9.598844408820456309 ) ) ;
#8616=CARTESIAN_POINT ( 'NONE',  ( -13.14518615778179189, 37.42812500108393436, 5.444914386472304635 ) ) ;
#8635=CARTESIAN_POINT ( 'NONE',  ( 0.000000000000000000, 0.000000000000000000, 0.000000000000000000 ) ) ;
#8653=CARTESIAN_POINT ( 'NONE',  ( -8.049105076161786076E-16, 38.17226562608394147, -13.14518615778179544 ) ) ;
#8654=CARTESIAN_POINT ( 'NONE',  ( 5.622872871577878406, 37.37851562716787157, 13.57481594606304576 ) ) ;
#8657=AXIS2_PLACEMENT_3D ( 'NONE', #20894, #1377, #25028 ) ;
#8662=VECTOR ( 'NONE', #23751, 1000.000000000000000 ) ;
#8672=CARTESIAN_POINT ( 'NONE',  ( -9.295050272127046043, 40.45429687608393721, -9.295050272127046043 ) ) ;
#8678=AXIS2_PLACEMENT_3D ( 'NONE', #2311, #2021, #10968 ) ;
#8680=CARTESIAN_POINT ( 'NONE',  ( 2.493653234604083739E-15, 35.74140625216787015, 13.57481594606304576 ) ) ;
#8687=AXIS2_PLACEMENT_3D ( 'NONE', #21022, #1503, #3492 ) ;
#8699=CARTESIAN_POINT ( 'NONE',  ( 2.414731522848535132E-15, 35.19570312608392726, 13.14518615778179544 ) ) ;
#8702=ORIENTED_EDGE ( 'NONE', *, *, #3595, .F. ) ;
#8718=( BOUNDED_CURVE ( )  B_SPLINE_CURVE ( 2, ( #27921, #23642, #12643, #25916, #8382, #19498, #10512, #25770, #4117 ),
 .UNSPECIFIED., .F., .F. ) 
 B_SPLINE_CURVE_WITH_KNOTS ( ( 3, 2, 2, 2, 3 ),
 ( 0.2291666666666665741, 0.2395833333333332316, 0.2499999999999998335, 0.2604166666666665186, 0.2708333333333330928 ),
 .UNSPECIFIED. ) 
 CURVE ( )  GEOMETRIC_REPRESENTATION_ITEM ( )  RATIONAL_B_SPLINE_CURVE ( ( 1.000000000000000666, 0.9238795325112861834, 1.000000000000000000, 0.9238795325112867385, 1.000000000000000000, 0.9238795325112867385, 1.000000000000000000, 0.9238795325112884038, 0.9999999999999983347 ) ) 
 REPRESENTATION_ITEM ( '' )  );
#8729=CARTESIAN_POINT ( 'NONE',  ( 5.622872871577780707, 33.70742187716788152, -13.57481594606313990 ) ) ;
#8740=CARTESIAN_POINT ( 'NONE',  ( -9.295050272127044266, 38.46992187608393721, 9.295050272127047819 ) ) ;
#8747=CARTESIAN_POINT ( 'NONE',  ( 2.414731522848535132E-15, 37.77539062608393294, 13.14518615778179544 ) ) ;
#8753=CARTESIAN_POINT ( 'NONE',  ( 5.622872871577878406, 36.48554687499999716, 13.57481594606304576 ) ) ;
#8754=CARTESIAN_POINT ( 'NONE',  ( 13.14518615778179900, 37.82500000108392868, -5.444914386472297529 ) ) ;
#8765=CYLINDRICAL_SURFACE ( 'NONE', #5762, 13.57481594606304576 ) ;
#8770=CARTESIAN_POINT ( 'NONE',  ( -9.598844408820454532, 36.43593750216787441, 9.598844408820459861 ) ) ;
#8790=CARTESIAN_POINT ( 'NONE',  ( -5.444914386472297529, 37.42812500108394147, -13.14518615778179900 ) ) ;
#8791=CARTESIAN_POINT ( 'NONE',  ( -13.57481594606304753, 37.87460937716787868, -5.622872871577873077 ) ) ;
#8802=CARTESIAN_POINT ( 'NONE',  ( -9.598844408820454532, 34.05468750216788010, 9.598844408820459861 ) ) ;
#8803=EDGE_CURVE ( 'NONE', #4431, #20608, #8344, .T. ) ;
#8812=CARTESIAN_POINT ( 'NONE',  ( 13.14518615778179544, 37.77539062608393294, -1.609821015232357215E-15 ) ) ;
#8816=CYLINDRICAL_SURFACE ( 'NONE', #24251, 13.57481594606304576 ) ;
#8834=CARTESIAN_POINT ( 'NONE',  ( 1.662435489736055892E-15, 40.99999999999999289, 13.57481594606304576 ) ) ;
#8841=CARTESIAN_POINT ( 'NONE',  ( 9.295050272127046043, 35.49335937608393010, -9.295050272127046043 ) ) ;
#8855=LINE ( 'NONE', #2029, #4418 ) ;
#8870=CARTESIAN_POINT ( 'NONE',  ( 9.598844408820459861, 33.45937500216787441, 9.598844408820456309 ) ) ;
#8882=CARTESIAN_POINT ( 'NONE',  ( 13.14518615778179900, 38.81718750108393579, -5.444914386472297529 ) ) ;
#8885=( BOUNDED_CURVE ( )  B_SPLINE_CURVE ( 2, ( #7892, #12288, #23011, #19143, #16585, #27848, #16727, #5909, #3899 ),
 .UNSPECIFIED., .F., .F. ) 
 B_SPLINE_CURVE_WITH_KNOTS ( ( 3, 2, 2, 2, 3 ),
 ( 0.6041666666666668517, 0.6145833333333334814, 0.6250000000000001110, 0.6354166666666667407, 0.6458333333333333703 ),
 .UNSPECIFIED. ) 
 CURVE ( )  GEOMETRIC_REPRESENTATION_ITEM ( )  RATIONAL_B_SPLINE_CURVE ( ( 0.9999999999999983347, 0.9238795325112884038, 1.000000000000000000, 0.9238795325112867385, 1.000000000000000000, 0.9238795325112867385, 1.000000000000000000, 0.9238795325112867385, 1.000000000000000000 ) ) 
 REPRESENTATION_ITEM ( '' )  );
#8889=CARTESIAN_POINT ( 'NONE',  ( -5.444914386472297529, 36.63437500108393863, -13.14518615778179722 ) ) ;
#8891=AXIS2_PLACEMENT_3D ( 'NONE', #21937, #2553, #6950 ) ;
#8896=CARTESIAN_POINT ( 'NONE',  ( 9.598844408820459861, 35.74140624999999716, 9.598844408820456309 ) ) ;
#8897=CARTESIAN_POINT ( 'NONE',  ( 13.14518615778179900, 37.72578125108393721, 5.444914386472293977 ) ) ;
#8911=CARTESIAN_POINT ( 'NONE',  ( -9.598844408820458085, 36.23750000216787726, -9.598844408820458085 ) ) ;
#8913=( NAMED_UNIT ( * ) SI_UNIT ( $, .STERADIAN. ) SOLID_ANGLE_UNIT ( ) );
#8932=( BOUNDED_CURVE ( )  B_SPLINE_CURVE ( 2, ( #9941, #12206, #14765, #4101, #23348 ),
 .UNSPECIFIED., .F., .F. ) 
 B_SPLINE_CURVE_WITH_KNOTS ( ( 3, 2, 3 ),
 ( 0.000000000000000000, 0.01041666666666679446, 0.02083333333333358892 ),
 .UNSPECIFIED. ) 
 CURVE ( )  GEOMETRIC_REPRESENTATION_ITEM ( )  RATIONAL_B_SPLINE_CURVE ( ( 1.000000000000000000, 0.9238795325112867385, 1.000000000000000000, 0.9238795325112848511, 1.000000000000001776 ) ) 
 REPRESENTATION_ITEM ( '' )  );
#8933=CARTESIAN_POINT ( 'NONE',  ( -8.049105076161786076E-16, 36.58476562608393579, -13.14518615778179544 ) ) ;
#8934=CARTESIAN_POINT ( 'NONE',  ( 9.598844408820459861, 38.22187500216787015, 9.598844408820456309 ) ) ;
#8944=CYLINDRICAL_SURFACE ( 'NONE', #22470, 13.57481594606304576 ) ;
#8954=CARTESIAN_POINT ( 'NONE',  ( 13.14518615778179900, 37.03125000108393294, -5.444914386472297529 ) ) ;
#8958=CARTESIAN_POINT ( 'NONE',  ( 13.57481594606304576, 39.01562500000000000, -1.662435489736055892E-15 ) ) ;
#8964=CARTESIAN_POINT ( 'NONE',  ( -8.312177448680279460E-16, 36.83281249999999574, -13.57481594606304576 ) ) ;
#8985=CARTESIAN_POINT ( 'NONE',  ( 9.295050272127047819, 35.29492187608393294, 9.295050272127046043 ) ) ;
#8989=VERTEX_POINT ( 'NONE', #18224 ) ;
#9027=EDGE_CURVE ( 'NONE', #16597, #23528, #11080, .T. ) ;
#9031=CARTESIAN_POINT ( 'NONE',  ( 9.295050272127047819, 40.25585937608393294, 9.295050272127046043 ) ) ;
#9036=CARTESIAN_POINT ( 'NONE',  ( -13.14518615778179189, 38.42031250108393436, 5.444914386472304635 ) ) ;
#9042=CARTESIAN_POINT ( 'NONE',  ( -13.57481594606304576, 36.23749999999999005, 0.000000000000000000 ) ) ;
#9043=CARTESIAN_POINT ( 'NONE',  ( -5.444914386472297529, 37.22968750108393721, -13.14518615778179900 ) ) ;
#9070=CARTESIAN_POINT ( 'NONE',  ( 2.493653234604083739E-15, 33.26093749999999716, 13.57481594606304576 ) ) ;
#9076=CARTESIAN_POINT ( 'NONE',  ( -13.14518615778179900, 38.32109375108394289, -5.444914386472297529 ) ) ;
#9077=CARTESIAN_POINT ( 'NONE',  ( -13.57481594606304576, 37.18007812716787441, 5.622872871577880183 ) ) ;
#9098=CARTESIAN_POINT ( 'NONE',  ( -13.14518615778179189, 37.42812500108393436, 5.444914386472304635 ) ) ;
#9117=ORIENTED_EDGE ( 'NONE', *, *, #7591, .T. ) ;
#9125=CARTESIAN_POINT ( 'NONE',  ( 5.444914386472302859, 32.07031250108393294, 13.14518615778179189 ) ) ;
#9126=CARTESIAN_POINT ( 'NONE',  ( 9.598844408820456309, 36.83281250216787583, -9.598844408820458085 ) ) ;
#9152=EDGE_CURVE ( 'NONE', #23528, #4431, #3234, .T. ) ;
#9170=CARTESIAN_POINT ( 'NONE',  ( -5.444914386472297529, 35.04687500108393294, -13.14518615778179900 ) ) ;
#9176=CARTESIAN_POINT ( 'NONE',  ( 13.14518615778179722, 36.43593750108394147, -5.444914386472297529 ) ) ;
#9181=CARTESIAN_POINT ( 'NONE',  ( -5.622872871577873077, 33.21132812499999432, 13.57481594606304753 ) ) ;
#9182=CARTESIAN_POINT ( 'NONE',  ( -13.14518615778179900, 34.15390625108393863, -5.444914386472297529 ) ) ;
#9195=CARTESIAN_POINT ( 'NONE',  ( -9.598844408820454532, 34.84843750216787583, 9.598844408820459861 ) ) ;
#9197=SHAPE_REPRESENTATION_RELATIONSHIP ( 'NONE' , 'NONE' ,  #19878, #15807 ) ;
#9217=CARTESIAN_POINT ( 'NONE',  ( -8.049105076161786076E-16, 35.79101562608394005, -13.14518615778179544 ) ) ;
#9218=CARTESIAN_POINT ( 'NONE',  ( 13.57481594606304753, 37.57695312716787583, -5.622872871577873077 ) ) ;
#9229=CARTESIAN_POINT ( 'NONE',  ( -13.57481594606304398, 31.62382812716787228, 5.622872871577880183 ) ) ;
#9239=CARTESIAN_POINT ( 'NONE',  ( 2.414731522848535132E-15, 35.19570312608392726, 13.14518615778179544 ) ) ;
#9242=CARTESIAN_POINT ( 'NONE',  ( 13.57481594606304931, 38.96601562499999005, 5.622872871577868636 ) ) ;
#9244=ADVANCED_FACE ( 'NONE', ( #22932 ), #12618, .F. ) ;
#9264=CARTESIAN_POINT ( 'NONE',  ( -13.14518615778179722, 34.15390625108393863, -5.444914386472297529 ) ) ;
#9304=CARTESIAN_POINT ( 'NONE',  ( 13.14518615778179900, 35.64218750108393152, -5.444914386472297529 ) ) ;
#9310=CARTESIAN_POINT ( 'NONE',  ( 5.444914386472297529, 38.12265625108393863, -13.14518615778179722 ) ) ;
#9316=CARTESIAN_POINT ( 'NONE',  ( 3.878385297391210518, 32.03609435653363136, -13.57481594606304576 ) ) ;
#9317=CARTESIAN_POINT ( 'NONE',  ( 9.295050272127046043, 33.11210937608393579, -9.295050272127046043 ) ) ;
#9350=CARTESIAN_POINT ( 'NONE',  ( 2.493653234604083739E-15, 34.94765625216787441, 13.57481594606304576 ) ) ;
#9355=CARTESIAN_POINT ( 'NONE',  ( -13.14518615778179900, 34.35234375108393579, -5.444914386472297529 ) ) ;
#9356=CARTESIAN_POINT ( 'NONE',  ( -9.598844408820458085, 33.85625000216787583, -9.598844408820458085 ) ) ;
#9374=CARTESIAN_POINT ( 'NONE',  ( 5.444914386472302859, 36.83281250108392868, 13.14518615778179189 ) ) ;
#9377=CARTESIAN_POINT ( 'NONE',  ( -9.598844408820454532, 38.02343750216788010, 9.598844408820459861 ) ) ;
#9383=DIRECTION ( 'NONE',  ( 0.000000000000000000, 0.000000000000000000, -1.000000000000000000 ) ) ;
#9395=ORIENTED_EDGE ( 'NONE', *, *, #13660, .T. ) ;
#9402=CARTESIAN_POINT ( 'NONE',  ( 9.295050272127047819, 32.11992187608393579, 9.295050272127046043 ) ) ;
#9445=CARTESIAN_POINT ( 'NONE',  ( 9.295050272127046043, 37.27929687608394005, -9.295050272127046043 ) ) ;
#9451=CARTESIAN_POINT ( 'NONE',  ( 5.444914386472297529, 34.94765625108394147, -13.14518615778179722 ) ) ;
#9457=CARTESIAN_POINT ( 'NONE',  ( 13.57481594606304576, 33.45937499999999432, -1.662435489736055892E-15 ) ) ;
#9458=CARTESIAN_POINT ( 'NONE',  ( -13.14518615778179900, 33.36015625108393579, -5.444914386472297529 ) ) ;
#9494=CARTESIAN_POINT ( 'NONE',  ( -8.049105076161786076E-16, 32.61601562608393579, -13.14518615778179544 ) ) ;
#9495=CARTESIAN_POINT ( 'NONE',  ( 5.622872871577878406, 33.40976562716787157, 13.57481594606304576 ) ) ;
#9509=DIRECTION ( 'NONE',  ( 0.000000000000000000, 0.000000000000000000, -1.000000000000000000 ) ) ;
#9511=EDGE_CURVE ( 'NONE', #5570, #10432, #12889, .T. ) ;
#9521=CARTESIAN_POINT ( 'NONE',  ( 2.414731522848535132E-15, 34.40195312608393152, 13.14518615778179544 ) ) ;
#9525=CARTESIAN_POINT ( 'NONE',  ( -5.622872871577782483, 35.29492187499999289, -13.57481594606313990 ) ) ;
#9535=( GEOMETRIC_REPRESENTATION_CONTEXT ( 3 ) GLOBAL_UNCERTAINTY_ASSIGNED_CONTEXT ( ( #4715 ) ) GLOBAL_UNIT_ASSIGNED_CONTEXT ( ( #4934, #22461, #661 ) ) REPRESENTATION_CONTEXT ( 'NONE', 'WORKASPACE' ) );
#9549=CARTESIAN_POINT ( 'NONE',  ( -9.295050272127044266, 32.71523437608393436, 9.295050272127047819 ) ) ;
#9564=DIRECTION ( 'NONE',  ( -0.000000000000000000, -1.000000000000000000, -0.000000000000000000 ) ) ;
#9566=ORIENTED_EDGE ( 'NONE', *, *, #11740, .T. ) ;
#9588=CARTESIAN_POINT ( 'NONE',  ( -13.14518615778179189, 36.83281250108393579, 5.444914386472304635 ) ) ;
#9594=CARTESIAN_POINT ( 'NONE',  ( 5.444914386472302859, 34.65000000108393863, 13.14518615778179189 ) ) ;
#9601=AXIS2_PLACEMENT_3D ( 'NONE', #2339, #25987, #15129 ) ;
#9602=CARTESIAN_POINT ( 'NONE',  ( -5.622872871577873077, 34.50117187499999005, -13.57481594606304753 ) ) ;
#9603=CARTESIAN_POINT ( 'NONE',  ( 13.14518615778179900, 33.85625000108393579, -5.444914386472297529 ) ) ;
#9623=CARTESIAN_POINT ( 'NONE',  ( 0.000000000000000000, 40.99999999999999289, 0.000000000000000000 ) ) ;
#9629=CARTESIAN_POINT ( 'NONE',  ( 9.598844408820459861, 35.04687500216787299, 9.598844408820456309 ) ) ;
#9631=LINE ( 'NONE', #26757, #27917 ) ;
#9636=CARTESIAN_POINT ( 'NONE',  ( 9.295050272127046043, 34.10429687608393579, -9.295050272127046043 ) ) ;
#9637=CARTESIAN_POINT ( 'NONE',  ( -13.57481594606304753, 34.69960937716787441, -5.622872871577873077 ) ) ;
#9657=CARTESIAN_POINT ( 'NONE',  ( -13.57481594606304753, 33.01289062499999716, -5.622872871577872189 ) ) ;
#9659=CARTESIAN_POINT ( 'NONE',  ( 2.414731522848535132E-15, 32.02070312608393010, 13.14518615778179544 ) ) ;
#9667=EDGE_CURVE ( 'NONE', #24795, #14317, #17790, .T. ) ;
#9692=CARTESIAN_POINT ( 'NONE',  ( 13.14518615778179722, 32.26875000108393721, -5.444914386472297529 ) ) ;
#9706=CARTESIAN_POINT ( 'NONE',  ( 13.57481594606304576, 39.80937499999999574, -1.662435489736055892E-15 ) ) ;
#9709=AXIS2_PLACEMENT_3D ( 'NONE', #23167, #3356, #12028 ) ;
#9718=EDGE_LOOP ( 'NONE', ( #27607, #14326 ) ) ;
#9730=CARTESIAN_POINT ( 'NONE',  ( -9.295050272127044266, 35.29492187608393294, 9.295050272127047819 ) ) ;
#9733=CARTESIAN_POINT ( 'NONE',  ( 13.57481594606304931, 32.61601562499999574, 5.622872871577868636 ) ) ;
#9736=CARTESIAN_POINT ( 'NONE',  ( -9.295050272127046043, 33.50898437608393010, -9.295050272127046043 ) ) ;
#9738=CARTESIAN_POINT ( 'NONE',  ( -5.622872871577920151, 36.08867187500000284, -13.57481594606300135 ) ) ;
#9741=CARTESIAN_POINT ( 'NONE',  ( 13.57481594606304931, 34.99726562500000426, 5.622872871577869525 ) ) ;
#9742=CARTESIAN_POINT ( 'NONE',  ( 13.14518615778179544, 34.60039062608392868, -1.609821015232357215E-15 ) ) ;
#9757=ORIENTED_EDGE ( 'NONE', *, *, #8291, .F. ) ;
#9769=CARTESIAN_POINT ( 'NONE',  ( 5.622872871578015186, 34.99726562716787015, 13.57481594606290543 ) ) ;
#9776=CARTESIAN_POINT ( 'NONE',  ( -9.295050272127044266, 32.91367187608393152, 9.295050272127047819 ) ) ;
#9777=CARTESIAN_POINT ( 'NONE',  ( -13.57481594606304576, 35.54296875216788010, 0.000000000000000000 ) ) ;
#9798=CARTESIAN_POINT ( 'NONE',  ( -8.312177448680279460E-16, 32.86406249999999574, -13.57481594606304576 ) ) ;
#9800=CARTESIAN_POINT ( 'NONE',  ( 13.14518615778179900, 33.75703125108393010, 5.444914386472293977 ) ) ;
#9842=AXIS2_PLACEMENT_3D ( 'NONE', #22049, #26468, #6369 ) ;
#9869=CARTESIAN_POINT ( 'NONE',  ( 5.444914386472302859, 33.85625000108393579, 13.14518615778179189 ) ) ;
#9873=CARTESIAN_POINT ( 'NONE',  ( 5.622872871577796694, 39.26367187716788010, -13.57481594606312036 ) ) ;
#9875=CARTESIAN_POINT ( 'NONE',  ( -9.295050272127044266, 35.29492187608393294, 9.295050272127047819 ) ) ;
#9889=CARTESIAN_POINT ( 'NONE',  ( -8.312177448680279460E-16, 33.65781249999999147, -13.57481594606304576 ) ) ;
#9908=CARTESIAN_POINT ( 'NONE',  ( 5.444914386472302859, 33.06250000108393294, 13.14518615778179189 ) ) ;
#9909=CARTESIAN_POINT ( 'NONE',  ( -13.57481594606304576, 33.16171875216787868, 0.000000000000000000 ) ) ;
#9928=VERTEX_POINT ( 'NONE', #859 ) ;
#9931=CARTESIAN_POINT ( 'NONE',  ( -9.295050272127046043, 34.10429687608393579, -9.295050272127046043 ) ) ;
#9941=CARTESIAN_POINT ( 'NONE',  ( -13.57481594606304576, 40.99999999999999289, 0.000000000000000000 ) ) ;
#9961=( BOUNDED_CURVE ( )  B_SPLINE_CURVE ( 2, ( #16065, #11638, #20924, #1129, #5679, #5254, #23061, #22646, #7518 ),
 .UNSPECIFIED., .F., .F. ) 
 B_SPLINE_CURVE_WITH_KNOTS ( ( 3, 2, 2, 2, 3 ),
 ( 0.02083333333333358892, 0.03125000000000020123, 0.04166666666666681007, 0.05208333333333342585, 0.06250000000000004163 ),
 .UNSPECIFIED. ) 
 CURVE ( )  GEOMETRIC_REPRESENTATION_ITEM ( )  RATIONAL_B_SPLINE_CURVE ( ( 0.9999999999999981126, 0.9238795325112886259, 1.000000000000000000, 0.9238795325112867385, 1.000000000000000000, 0.9238795325112867385, 1.000000000000000000, 0.9238795325112864054, 1.000000000000000222 ) ) 
 REPRESENTATION_ITEM ( '' )  );
#9975=( GEOMETRIC_REPRESENTATION_CONTEXT ( 3 ) GLOBAL_UNCERTAINTY_ASSIGNED_CONTEXT ( ( #15526 ) ) GLOBAL_UNIT_ASSIGNED_CONTEXT ( ( #1949, #26309, #8913 ) ) REPRESENTATION_CONTEXT ( 'NONE', 'WORKASPACE' ) );
#10001=CARTESIAN_POINT ( 'NONE',  ( -13.14518615778179900, 34.35234375108393579, -5.444914386472297529 ) ) ;
#10008=CARTESIAN_POINT ( 'NONE',  ( 6.944426393311537993, 31.75150625057403175, -11.16113171639042356 ) ) ;
#10019=EDGE_CURVE ( 'NONE', #10042, #7430, #8932, .T. ) ;
#10033=CARTESIAN_POINT ( 'NONE',  ( 2.493653234604083739E-15, 40.40468749999999432, 13.57481594606304576 ) ) ;
#10042=VERTEX_POINT ( 'NONE', #25483 ) ;
#10046=CARTESIAN_POINT ( 'NONE',  ( 5.622872871577871301, 39.16445312499999432, -13.57481594606304753 ) ) ;
#10047=CARTESIAN_POINT ( 'NONE',  ( -8.049105076161786076E-16, 39.56132812608393579, -13.14518615778179544 ) ) ;
#10076=CARTESIAN_POINT ( 'NONE',  ( 13.57481594606304931, 33.40976562499999858, 5.622872871577868636 ) ) ;
#10082=CARTESIAN_POINT ( 'NONE',  ( -8.312177448680279460E-16, 39.31328125216787583, -13.57481594606304576 ) ) ;
#10092=CARTESIAN_POINT ( 'NONE',  ( 0.000000000000000000, 40.99999999999999289, -13.57481594606304576 ) ) ;
#10122=CARTESIAN_POINT ( 'NONE',  ( 9.295050272127047819, 39.26367187608393294, 9.295050272127046043 ) ) ;
#10127=ORIENTED_EDGE ( 'NONE', *, *, #9511, .F. ) ;
#10131=CARTESIAN_POINT ( 'NONE',  ( 5.444914386472302859, 32.26875000108393721, 13.14518615778179189 ) ) ;
#10136=CARTESIAN_POINT ( 'NONE',  ( 9.598844408820459861, 39.01562500216787299, 9.598844408820456309 ) ) ;
#10144=ORIENTED_EDGE ( 'NONE', *, *, #13111, .F. ) ;
#10156=EDGE_CURVE ( 'NONE', #58, #18296, #5870, .T. ) ;
#10167=CARTESIAN_POINT ( 'NONE',  ( -5.444914386472297529, 39.80937500108393579, -13.14518615778179722 ) ) ;
#10172=EDGE_CURVE ( 'NONE', #10042, #637, #5420, .T. ) ;
#10174=CARTESIAN_POINT ( 'NONE',  ( 13.57481594606304753, 38.27148437500000711, -5.622872871577873077 ) ) ;
#10175=CARTESIAN_POINT ( 'NONE',  ( -5.622872871577873077, 31.72304687716787441, 13.57481594606304753 ) ) ;
#10218=CARTESIAN_POINT ( 'NONE',  ( -13.57481594606304576, 40.65273437608393436, 0.000000000000000000 ) ) ;
#10223=VERTEX_POINT ( 'NONE', #2102 ) ;
#10251=AXIS2_PLACEMENT_3D ( 'NONE', #1308, #9564, #16113 ) ;
#10261=CARTESIAN_POINT ( 'NONE',  ( 2.414731522848535132E-15, 39.95820312608393010, 13.14518615778179544 ) ) ;
#10272=CARTESIAN_POINT ( 'NONE',  ( 13.14518615778179544, 34.00507812608393721, -1.609821015232357215E-15 ) ) ;
#10285=EDGE_CURVE ( 'NONE', #3669, #1494, #17193, .T. ) ;
#10288=ORIENTED_EDGE ( 'NONE', *, *, #1313, .T. ) ;
#10304=CARTESIAN_POINT ( 'NONE',  ( -9.598844408820454532, 40.30546874999999574, 9.598844408820459861 ) ) ;
#10307=CARTESIAN_POINT ( 'NONE',  ( -5.444914386472297529, 40.60312500108393863, -13.14518615778179722 ) ) ;
#10313=CARTESIAN_POINT ( 'NONE',  ( 2.493653234604083739E-15, 39.61093749999999147, 13.57481594606304576 ) ) ;
#10314=CARTESIAN_POINT ( 'NONE',  ( -9.295050272127044266, 39.85898437608393152, 9.295050272127047819 ) ) ;
#10326=FACE_OUTER_BOUND ( 'NONE', #21252, .T. ) ;
#10336=CARTESIAN_POINT ( 'NONE',  ( -8.312177448680279460E-16, 32.16953125216787157, -13.57481594606304576 ) ) ;
#10337=VERTEX_POINT ( 'NONE', #15469 ) ;
#10355=CARTESIAN_POINT ( 'NONE',  ( 5.444914386472302859, 39.41250000108393436, 13.14518615778179189 ) ) ;
#10366=EDGE_LOOP ( 'NONE', ( #24879, #17415, #7465, #2784 ) ) ;
#10370=CARTESIAN_POINT ( 'NONE',  ( 3.878384841496545388, 31.34156311272377238, -13.57481594606304753 ) ) ;
#10377=CARTESIAN_POINT ( 'NONE',  ( -13.14518615778179900, 38.91640625108393436, -5.444914386472297529 ) ) ;
#10407=CARTESIAN_POINT ( 'NONE',  ( 9.295050272127046043, 40.25585937608393294, -9.295050272127046043 ) ) ;
#10419=CARTESIAN_POINT ( 'NONE',  ( 9.295050272127047819, 32.31835937608393294, 9.295050272127046043 ) ) ;
#10425=CARTESIAN_POINT ( 'NONE',  ( 9.295050272127047819, 33.11210937608393579, 9.295050272127046043 ) ) ;
#10432=VERTEX_POINT ( 'NONE', #3507 ) ;
#10449=CARTESIAN_POINT ( 'NONE',  ( -5.444914386472299306, 34.35234375108392868, 13.14518615778179722 ) ) ;
#10455=VECTOR ( 'NONE', #1722, 1000.000000000000000 ) ;
#10461=CARTESIAN_POINT ( 'NONE',  ( -13.57481594606304576, 40.20624999999999005, 0.000000000000000000 ) ) ;
#10462=CARTESIAN_POINT ( 'NONE',  ( -5.622872871577873077, 32.21914062716787441, -13.57481594606304753 ) ) ;
#10479=ORIENTED_EDGE ( 'NONE', *, *, #24799, .T. ) ;
#10482=ORIENTED_EDGE ( 'NONE', *, *, #13111, .T. ) ;
#10500=CARTESIAN_POINT ( 'NONE',  ( 13.14518615778179900, 39.51171875108392584, 5.444914386472293977 ) ) ;
#10501=CARTESIAN_POINT ( 'NONE',  ( 5.622872871577878406, 39.75976562716787299, 13.57481594606304576 ) ) ;
#10512=CARTESIAN_POINT ( 'NONE',  ( -9.598844408820458085, 38.51953124999999289, -9.598844408820458085 ) ) ;
#10546=CARTESIAN_POINT ( 'NONE',  ( -9.295050272127046043, 38.07304687608393579, -9.295050272127046043 ) ) ;
#10552=ORIENTED_EDGE ( 'NONE', *, *, #11729, .T. ) ;
#10568=CARTESIAN_POINT ( 'NONE',  ( -13.14518615778179189, 32.86406250108393579, 5.444914386472304635 ) ) ;
#10572=CARTESIAN_POINT ( 'NONE',  ( -13.57481594606304753, 37.08085937716787583, -5.622872871577872189 ) ) ;
#10591=CARTESIAN_POINT ( 'NONE',  ( 13.14518615778179900, 38.71796875108393721, 5.444914386472293977 ) ) ;
#10596=CARTESIAN_POINT ( 'NONE',  ( -5.444914386472299306, 40.10703125108393152, 13.14518615778179722 ) ) ;
#10603=CARTESIAN_POINT ( 'NONE',  ( -5.622872871577873077, 39.56132812499999574, 13.57481594606304753 ) ) ;
#10604=CARTESIAN_POINT ( 'NONE',  ( 5.622872871577871301, 32.11992187716787583, -13.57481594606304753 ) ) ;
#10612=CARTESIAN_POINT ( 'NONE',  ( -8.312177448680279460E-16, 38.51953125216787299, -13.57481594606304576 ) ) ;
#10622=ORIENTED_EDGE ( 'NONE', *, *, #15237, .T. ) ;
#10633=CARTESIAN_POINT ( 'NONE',  ( 9.598844408820459861, 33.36015624999999574, 9.598844408820456309 ) ) ;
#10638=CARTESIAN_POINT ( 'NONE',  ( -5.444914386472299306, 38.51953125108393294, 13.14518615778179722 ) ) ;
#10655=CARTESIAN_POINT ( 'NONE',  ( -9.295050272127046043, 38.07304687608393579, -9.295050272127046043 ) ) ;
#10682=CARTESIAN_POINT ( 'NONE',  ( 5.444914386472302859, 36.03906250108393294, 13.14518615778179189 ) ) ;
#10713=FACE_OUTER_BOUND ( 'NONE', #18311, .T. ) ;
#10727=CARTESIAN_POINT ( 'NONE',  ( 13.14518615778179544, 37.97382812608393721, -1.609821015232357215E-15 ) ) ;
#10739=CARTESIAN_POINT ( 'NONE',  ( 13.57481594606304576, 38.22187499999999716, -1.662435489736055892E-15 ) ) ;
#10740=CARTESIAN_POINT ( 'NONE',  ( 9.295050272127047819, 36.08867187608392868, 9.295050272127046043 ) ) ;
#10774=CARTESIAN_POINT ( 'NONE',  ( 0.000000000000000000, 40.99999999999999289, 0.000000000000000000 ) ) ;
#10775=CARTESIAN_POINT ( 'NONE',  ( 2.414731522848535132E-15, 36.98164062608393721, 13.14518615778179544 ) ) ;
#10776=CARTESIAN_POINT ( 'NONE',  ( -9.598844408820458085, 36.23750000216787726, -9.598844408820458085 ) ) ;
#10781=B_SPLINE_CURVE_WITH_KNOTS ( 'NONE', 3,
 ( #20176, #3212, #4932, #22605 ),
 .UNSPECIFIED., .F., .F.,
 ( 4, 4 ),
 ( 0.000000000000000000, 1.000000000000000000 ),
 .UNSPECIFIED. ) ;
#10786=CARTESIAN_POINT ( 'NONE',  ( -13.57481594606304753, 33.90585937716787868, -5.622872871577872189 ) ) ;
#10793=CARTESIAN_POINT ( 'NONE',  ( -9.295050272127044266, 39.85898437608393152, 9.295050272127047819 ) ) ;
#10800=CARTESIAN_POINT ( 'NONE',  ( 7.171391131791534868, 31.93754143773660203, -11.52591762960188149 ) ) ;
#10808=ORIENTED_EDGE ( 'NONE', *, *, #9152, .T. ) ;
#10814=ORIENTED_EDGE ( 'NONE', *, *, #8099, .F. ) ;
#10818=CARTESIAN_POINT ( 'NONE',  ( -13.14518615778179544, 37.37851562608393863, 0.000000000000000000 ) ) ;
#10838=ORIENTED_EDGE ( 'NONE', *, *, #24988, .T. ) ;
#10845=CYLINDRICAL_SURFACE ( 'NONE', #14255, 13.57481594606304576 ) ;
#10859=CARTESIAN_POINT ( 'NONE',  ( 13.57481594606304753, 37.47773437500001137, -5.622872871577873966 ) ) ;
#10863=CARTESIAN_POINT ( 'NONE',  ( 5.444914386472297529, 39.71015625108393010, -13.14518615778179900 ) ) ;
#10871=CARTESIAN_POINT ( 'NONE',  ( 5.444914386472302859, 37.03125000108393294, 13.14518615778179189 ) ) ;
#10872=CARTESIAN_POINT ( 'NONE',  ( -13.57481594606304753, 39.46210937716787726, -5.622872871577872189 ) ) ;
#10880=CARTESIAN_POINT ( 'NONE',  ( 5.622872871577878406, 38.07304687499998863, 13.57481594606304576 ) ) ;
#10881=CARTESIAN_POINT ( 'NONE',  ( -9.295050272127046043, 38.07304687608393579, -9.295050272127046043 ) ) ;
#10902=LINE ( 'NONE', #6915, #8662 ) ;
#10910=DIRECTION ( 'NONE',  ( 0.000000000000000000, 0.000000000000000000, 1.000000000000000000 ) ) ;
#10916=( BOUNDED_SURFACE ( )  B_SPLINE_SURFACE ( 1, 2, ( 
 ( #23080, #16922, #1838, #25622, #3827, #8096, #25489, #5967, #17200, #6104, #21357, #10501, #14771, #19208, #25760, #6242, #4107, #3555, #12212, #20941, #10082, #18794, #27501, #7956, #16655, #5834, #14502, #23219, #17345, #4811, #13470, #21922, #22196, #23905, #21633, #26622, #2397, #15625, #2675, #4385, #13183, #6647, #8934, #13042, #17911, #23767, #20057, #11336, #536, #8791, #19488, #2531, #6512, #11055, #24327, #9218, #21777, #17482, #24190, #8654, #248, #2256, #395, #9077, #26041, #24049, #17772, #15187, #4524, #19764, #28186, #26476, #15049, #10918, #11193, #6932, #19627, #4243, #19912, #15333, #12903, #2109, #10776, #109, #26181, #17623, #26330, #6790, #15475, #4669, #13331, #22057, #1110, #22340, #22625, #22904, #9777, #5378, #25037, #11901, #18195, #5519, #2810, #828, #18623, #15764, #26762, #16043, #5094, #11616, #7069, #18485, #20487, #9637, #26906, #3096, #3367, #7644, #27193, #968, #24471, #4956, #14186, #20196, #16337, #24897, #11479, #14047, #681, #24616, #9356, #12038, #20625, #24753, #5234, #22481, #13617, #18049, #7204, #9495, #20762, #1246, #7352, #15899, #9909, #13756, #2946, #20341, #18342, #13900, #11763, #27047, #7495, #16191, #22768, #3233, #1523, #5656, #5931, #16885, #27327, #1386, #25451, #10462, #14462, #10604, #7786, #14599, #3790, #25308, #27461, #19170, #6204, #10175, #17018, #23317, #27735, #20904, #14321, #14874, #12448, #27871, #7919 ),
 ( #16615, #21175, #18885, #1655, #5796, #1935, #16473, #4071, #23589, #12733, #21039, #3513, #14733, #18758, #10314, #8334, #25721, #23181, #27594, #8195, #10047, #19022, #3655, #12589, #21313, #12318, #8055, #1797, #16750, #25584, #6067, #12174, #21457, #25168, #23453, #3931, #23042, #12865, #11155, #6754, #19590, #13288, #22017, #17735, #15150, #356, #4772, #23868, #19727, #212, #10881, #24012, #24153, #73, #4630, #8754, #26004, #8897, #26145, #24291, #15295, #4346, #6896, #8616, #19871, #22160, #21595, #9043, #26437, #6610, #15583, #28149, #25866, #2638, #4490, #13432, #19311, #17304, #17446, #13147, #21884, #6475, #28011, #8476, #17165, #6337, #15011, #13002, #23732, #15438, #10740, #2359, #4206, #2070, #21741, #2217, #17587, #19450, #11014, #26292, #2494, #24860, #22303, #20302, #5341, #4919, #788, #26872, #15727, #14007, #20590, #13580, #27012, #22730, #2778, #3197, #7459, #11582, #11868, #1073, #9742, #7170, #18451, #25001, #15867, #16154, #24431, #17875, #2912, #9182, #27157, #26581, #7318, #7610, #16300, #9603, #5481, #14151, #22445, #22870, #7030, #5059, #11300, #20021, #11442, #9458, #20162, #18160, #501, #644, #9317, #18014, #26725, #24577, #13723, #16007, #24721, #5199, #13864, #22589, #3058, #11724, #18304, #20450, #932, #7886, #12284, #23007, #18725, #12143, #14290, #27293, #25134, #7750, #14431, #23147, #16581, #27423, #5761, #25273, #5624, #3622, #20732 ) ),
 .UNSPECIFIED., .F., .F., .F. ) 
 B_SPLINE_SURFACE_WITH_KNOTS ( ( 2, 2 ),
 ( 3, 2, 2, 2, 2, 2, 2, 2, 2, 2, 2, 2, 2, 2, 2, 2, 2, 2, 2, 2, 2, 2, 2, 2, 2, 2, 2, 2, 2, 2, 2, 2, 2, 2, 2, 2, 2, 2, 2, 2, 2, 2, 2, 2, 2, 2, 2, 2, 2, 2, 2, 2, 2, 2, 2, 2, 2, 2, 2, 2, 2, 2, 2, 2, 2, 2, 2, 2, 2, 2, 2, 2, 2, 2, 2, 2, 2, 2, 2, 2, 2, 2, 2, 2, 2, 2, 2, 2, 2, 2, 2, 3 ),
 ( 0.000000000000000000, 1.000000000000000000 ),
 ( 0.000000000000000000, 0.01041666666666666609, 0.02083333333333333218, 0.03125000000000000000, 0.04166666666666666435, 0.05208333333333333565, 0.06250000000000000000, 0.07291666666666667129, 0.08333333333333332871, 0.09375000000000000000, 0.1041666666666666713, 0.1145833333333333287, 0.1250000000000000000, 0.1354166666666666574, 0.1458333333333333426, 0.1562500000000000000, 0.1666666666666666574, 0.1770833333333333426, 0.1875000000000000000, 0.1979166666666666574, 0.2083333333333333426, 0.2187500000000000000, 0.2291666666666666574, 0.2395833333333333426, 0.2500000000000000000, 0.2604166666666666852, 0.2708333333333333148, 0.2812500000000000000, 0.2916666666666666852, 0.3020833333333333148, 0.3125000000000000000, 0.3229166666666666852, 0.3333333333333333148, 0.3437500000000000000, 0.3541666666666666852, 0.3645833333333333148, 0.3750000000000000000, 0.3854166666666666852, 0.3958333333333333148, 0.4062500000000000000, 0.4166666666666666852, 0.4270833333333333148, 0.4375000000000000000, 0.4479166666666666852, 0.4583333333333333148, 0.4687500000000000000, 0.4791666666666666852, 0.4895833333333333148, 0.5000000000000000000, 0.5104166666666666297, 0.5208333333333333703, 0.5312500000000000000, 0.5416666666666666297, 0.5520833333333333703, 0.5625000000000000000, 0.5729166666666666297, 0.5833333333333333703, 0.5937500000000000000, 0.6041666666666666297, 0.6145833333333333703, 0.6250000000000000000, 0.6354166666666666297, 0.6458333333333333703, 0.6562500000000000000, 0.6666666666666666297, 0.6770833333333333703, 0.6875000000000000000, 0.6979166666666666297, 0.7083333333333333703, 0.7187500000000000000, 0.7291666666666666297, 0.7395833333333333703, 0.7500000000000000000, 0.7604166666666666297, 0.7708333333333333703, 0.7812500000000000000, 0.7916666666666666297, 0.8020833333333333703, 0.8125000000000000000, 0.8229166666666666297, 0.8333333333333333703, 0.8437500000000000000, 0.8541666666666666297, 0.8645833333333333703, 0.8750000000000000000, 0.8854166666666666297, 0.8958333333333333703, 0.9062500000000000000, 0.9166666666666666297, 0.9270833333333333703, 0.9375000000000000000, 0.9448586970929392370 ),
 .UNSPECIFIED. ) 
 GEOMETRIC_REPRESENTATION_ITEM ( )  RATIONAL_B_SPLINE_SURFACE ( (
 ( 1.000000000000000000, 0.9238795325112867385, 1.000000000000000000, 0.9238795325112867385, 1.000000000000000000, 0.9238795325112867385, 1.000000000000000000, 0.9238795325112867385, 1.000000000000000000, 0.9238795325112867385, 1.000000000000000000, 0.9238795325112867385, 1.000000000000000000, 0.9238795325112867385, 1.000000000000000000, 0.9238795325112867385, 1.000000000000000000, 0.9238795325112867385, 1.000000000000000000, 0.9238795325112867385, 1.000000000000000000, 0.9238795325112867385, 1.000000000000000000, 0.9238795325112867385, 1.000000000000000000, 0.9238795325112867385, 1.000000000000000000, 0.9238795325112867385, 1.000000000000000000, 0.9238795325112867385, 1.000000000000000000, 0.9238795325112867385, 1.000000000000000000, 0.9238795325112867385, 1.000000000000000000, 0.9238795325112867385, 1.000000000000000000, 0.9238795325112867385, 1.000000000000000000, 0.9238795325112867385, 1.000000000000000000, 0.9238795325112867385, 1.000000000000000000, 0.9238795325112867385, 1.000000000000000000, 0.9238795325112867385, 1.000000000000000000, 0.9238795325112867385, 1.000000000000000000, 0.9238795325112867385, 1.000000000000000000, 0.9238795325112867385, 1.000000000000000000, 0.9238795325112867385, 1.000000000000000000, 0.9238795325112867385, 1.000000000000000000, 0.9238795325112867385, 1.000000000000000000, 0.9238795325112867385, 1.000000000000000000, 0.9238795325112867385, 1.000000000000000000, 0.9238795325112867385, 1.000000000000000000, 0.9238795325112867385, 1.000000000000000000, 0.9238795325112867385, 1.000000000000000000, 0.9238795325112867385, 1.000000000000000000, 0.9238795325112867385, 1.000000000000000000, 0.9238795325112867385, 1.000000000000000000, 0.9238795325112867385, 1.000000000000000000, 0.9238795325112867385, 1.000000000000000000, 0.9238795325112867385, 1.000000000000000000, 0.9238795325112867385, 1.000000000000000000, 0.9238795325112867385, 1.000000000000000000, 0.9238795325112867385, 1.000000000000000000, 0.9238795325112867385, 1.000000000000000000, 0.9238795325112867385, 1.000000000000000000, 0.9238795325112867385, 1.000000000000000000, 0.9238795325112867385, 1.000000000000000000, 0.9238795325112867385, 1.000000000000000000, 0.9238795325112867385, 1.000000000000000000, 0.9238795325112867385, 1.000000000000000000, 0.9238795325112867385, 1.000000000000000000, 0.9238795325112867385, 1.000000000000000000, 0.9238795325112867385, 1.000000000000000000, 0.9238795325112867385, 1.000000000000000000, 0.9238795325112867385, 1.000000000000000000, 0.9238795325112867385, 1.000000000000000000, 0.9238795325112867385, 1.000000000000000000, 0.9238795325112867385, 1.000000000000000000, 0.9238795325112867385, 1.000000000000000000, 0.9238795325112867385, 1.000000000000000000, 0.9238795325112867385, 1.000000000000000000, 0.9238795325112867385, 1.000000000000000000, 0.9238795325112867385, 1.000000000000000000, 0.9238795325112867385, 1.000000000000000000, 0.9238795325112867385, 1.000000000000000000, 0.9238795325112867385, 1.000000000000000000, 0.9238795325112867385, 1.000000000000000000, 0.9238795325112867385, 1.000000000000000000, 0.9238795325112867385, 1.000000000000000000, 0.9238795325112867385, 1.000000000000000000, 0.9238795325112867385, 1.000000000000000000, 0.9238795325112867385, 1.000000000000000000, 0.9238795325112867385, 1.000000000000000000, 0.9238795325112867385, 1.000000000000000000, 0.9238795325112867385, 1.000000000000000000, 0.9238795325112867385, 1.000000000000000000, 0.9238795325112867385, 1.000000000000000000, 0.9238795325112867385, 1.000000000000000000, 0.9238795325112867385, 1.000000000000000000, 0.9238795325112867385, 1.000000000000000000, 0.9238795325112867385, 1.000000000000000000, 0.9238795325112867385, 1.000000000000000000, 0.9238795325112867385, 1.000000000000000000, 0.9238795325112867385, 1.000000000000000000, 0.9238795325112867385, 1.000000000000000000, 0.9238795325112867385, 1.000000000000000000, 0.9238795325112867385, 1.000000000000000000, 0.9238795325112867385, 1.000000000000000000, 0.9238795325112867385, 1.000000000000000000, 0.9238795325112867385, 1.000000000000000000, 0.9462258435690522607, 0.9684275710300105366),
 ( 1.000000000000000000, 0.9238795325112867385, 1.000000000000000000, 0.9238795325112867385, 1.000000000000000000, 0.9238795325112867385, 1.000000000000000000, 0.9238795325112867385, 1.000000000000000000, 0.9238795325112867385, 1.000000000000000000, 0.9238795325112867385, 1.000000000000000000, 0.9238795325112867385, 1.000000000000000000, 0.9238795325112867385, 1.000000000000000000, 0.9238795325112867385, 1.000000000000000000, 0.9238795325112867385, 1.000000000000000000, 0.9238795325112867385, 1.000000000000000000, 0.9238795325112867385, 1.000000000000000000, 0.9238795325112867385, 1.000000000000000000, 0.9238795325112867385, 1.000000000000000000, 0.9238795325112867385, 1.000000000000000000, 0.9238795325112867385, 1.000000000000000000, 0.9238795325112867385, 1.000000000000000000, 0.9238795325112867385, 1.000000000000000000, 0.9238795325112867385, 1.000000000000000000, 0.9238795325112867385, 1.000000000000000000, 0.9238795325112867385, 1.000000000000000000, 0.9238795325112867385, 1.000000000000000000, 0.9238795325112867385, 1.000000000000000000, 0.9238795325112867385, 1.000000000000000000, 0.9238795325112867385, 1.000000000000000000, 0.9238795325112867385, 1.000000000000000000, 0.9238795325112867385, 1.000000000000000000, 0.9238795325112867385, 1.000000000000000000, 0.9238795325112867385, 1.000000000000000000, 0.9238795325112867385, 1.000000000000000000, 0.9238795325112867385, 1.000000000000000000, 0.9238795325112867385, 1.000000000000000000, 0.9238795325112867385, 1.000000000000000000, 0.9238795325112867385, 1.000000000000000000, 0.9238795325112867385, 1.000000000000000000, 0.9238795325112867385, 1.000000000000000000, 0.9238795325112867385, 1.000000000000000000, 0.9238795325112867385, 1.000000000000000000, 0.9238795325112867385, 1.000000000000000000, 0.9238795325112867385, 1.000000000000000000, 0.9238795325112867385, 1.000000000000000000, 0.9238795325112867385, 1.000000000000000000, 0.9238795325112867385, 1.000000000000000000, 0.9238795325112867385, 1.000000000000000000, 0.9238795325112867385, 1.000000000000000000, 0.9238795325112867385, 1.000000000000000000, 0.9238795325112867385, 1.000000000000000000, 0.9238795325112867385, 1.000000000000000000, 0.9238795325112867385, 1.000000000000000000, 0.9238795325112867385, 1.000000000000000000, 0.9238795325112867385, 1.000000000000000000, 0.9238795325112867385, 1.000000000000000000, 0.9238795325112867385, 1.000000000000000000, 0.9238795325112867385, 1.000000000000000000, 0.9238795325112867385, 1.000000000000000000, 0.9238795325112867385, 1.000000000000000000, 0.9238795325112867385, 1.000000000000000000, 0.9238795325112867385, 1.000000000000000000, 0.9238795325112867385, 1.000000000000000000, 0.9238795325112867385, 1.000000000000000000, 0.9238795325112867385, 1.000000000000000000, 0.9238795325112867385, 1.000000000000000000, 0.9238795325112867385, 1.000000000000000000, 0.9238795325112867385, 1.000000000000000000, 0.9238795325112867385, 1.000000000000000000, 0.9238795325112867385, 1.000000000000000000, 0.9238795325112867385, 1.000000000000000000, 0.9238795325112867385, 1.000000000000000000, 0.9238795325112867385, 1.000000000000000000, 0.9238795325112867385, 1.000000000000000000, 0.9238795325112867385, 1.000000000000000000, 0.9238795325112867385, 1.000000000000000000, 0.9238795325112867385, 1.000000000000000000, 0.9238795325112867385, 1.000000000000000000, 0.9238795325112867385, 1.000000000000000000, 0.9238795325112867385, 1.000000000000000000, 0.9238795325112867385, 1.000000000000000000, 0.9238795325112867385, 1.000000000000000000, 0.9238795325112867385, 1.000000000000000000, 0.9238795325112867385, 1.000000000000000000, 0.9238795325112867385, 1.000000000000000000, 0.9238795325112867385, 1.000000000000000000, 0.9238795325112867385, 1.000000000000000000, 0.9238795325112867385, 1.000000000000000000, 0.9238795325112867385, 1.000000000000000000, 0.9238795325112867385, 1.000000000000000000, 0.9238795325112867385, 1.000000000000000000, 0.9238795325112867385, 1.000000000000000000, 0.9238795325112867385, 1.000000000000000000, 0.9238795325112867385, 1.000000000000000000, 0.9462258435690522607, 0.9684275710300105366) ) ) 
 REPRESENTATION_ITEM ( '' )  SURFACE ( )  );
#10917=CARTESIAN_POINT ( 'NONE',  ( -8.049105076161786076E-16, 37.37851562608393863, -13.14518615778179544 ) ) ;
#10918=CARTESIAN_POINT ( 'NONE',  ( 13.57481594606304931, 36.68398437716788152, 5.622872871577869525 ) ) ;
#10934=CARTESIAN_POINT ( 'NONE',  ( 9.295050272127046043, 39.46210937608393010, -9.295050272127046043 ) ) ;
#10944=ORIENTED_EDGE ( 'NONE', *, *, #4304, .F. ) ;
#10954=ORIENTED_EDGE ( 'NONE', *, *, #20222, .T. ) ;
#10962=CARTESIAN_POINT ( 'NONE',  ( 2.414731522848535132E-15, 36.78320312608393294, 13.14518615778179544 ) ) ;
#10968=DIRECTION ( 'NONE',  ( 0.000000000000000000, 0.000000000000000000, -1.000000000000000000 ) ) ;
#10974=FACE_OUTER_BOUND ( 'NONE', #20949, .T. ) ;
#10987=EDGE_CURVE ( 'NONE', #3669, #6267, #12713, .T. ) ;
#11001=CARTESIAN_POINT ( 'NONE',  ( -13.14518615778179189, 37.62656250108393863, 5.444914386472304635 ) ) ;
#11004=CARTESIAN_POINT ( 'NONE',  ( 9.598844408820456309, 38.32109374999999574, -9.598844408820458085 ) ) ;
#11007=CARTESIAN_POINT ( 'NONE',  ( 13.14518615778179722, 38.02343750108395426, -5.444914386472297529 ) ) ;
#11013=CARTESIAN_POINT ( 'NONE',  ( -9.598844408820458085, 36.93203124999999432, -9.598844408820458085 ) ) ;
#11014=CARTESIAN_POINT ( 'NONE',  ( -9.295050272127046043, 35.69179687608393436, -9.295050272127046043 ) ) ;
#11029=ADVANCED_FACE ( 'NONE', ( #17056 ), #10916, .F. ) ;
#11030=CARTESIAN_POINT ( 'NONE',  ( -8.312177448680279460E-16, 34.45156249999999432, -13.57481594606304576 ) ) ;
#11054=CARTESIAN_POINT ( 'NONE',  ( -9.295050272127044266, 36.88242187608393152, 9.295050272127047819 ) ) ;
#11055=CARTESIAN_POINT ( 'NONE',  ( 5.622872871577871301, 37.67617187716787441, -13.57481594606304753 ) ) ;
#11075=CARTESIAN_POINT ( 'NONE',  ( -9.295050272127044266, 35.09648437608392868, 9.295050272127047819 ) ) ;
#11080=( BOUNDED_CURVE ( )  B_SPLINE_CURVE ( 2, ( #3262, #2834, #9377, #16362, #7523, #16070, #24778, #24642, #852 ),
 .UNSPECIFIED., .F., .F. ) 
 B_SPLINE_CURVE_WITH_KNOTS ( ( 3, 2, 2, 2, 3 ),
 ( 0.2291666666666665741, 0.2395833333333332316, 0.2499999999999998335, 0.2604166666666665186, 0.2708333333333330928 ),
 .UNSPECIFIED. ) 
 CURVE ( )  GEOMETRIC_REPRESENTATION_ITEM ( )  RATIONAL_B_SPLINE_CURVE ( ( 1.000000000000000666, 0.9238795325112861834, 1.000000000000000000, 0.9238795325112867385, 1.000000000000000000, 0.9238795325112867385, 1.000000000000000000, 0.9238795325112884038, 0.9999999999999983347 ) ) 
 REPRESENTATION_ITEM ( '' )  );
#11082=CARTESIAN_POINT ( 'NONE',  ( -13.57481594606304398, 35.59257812716789715, 5.622872871577880183 ) ) ;
#11087=EDGE_LOOP ( 'NONE', ( #13227, #17769, #1317, #10479 ) ) ;
#11092=CARTESIAN_POINT ( 'NONE',  ( 13.57481594606304576, 34.25312499999999716, -1.662435489736055892E-15 ) ) ;
#11103=CARTESIAN_POINT ( 'NONE',  ( 9.295050272127047819, 36.88242187608393152, 9.295050272127046043 ) ) ;
#11140=CARTESIAN_POINT ( 'NONE',  ( -9.295050272127046043, 40.65273437608393436, -9.295050272127046043 ) ) ;
#11146=CARTESIAN_POINT ( 'NONE',  ( 13.14518615778179722, 38.81718750108393579, -5.444914386472297529 ) ) ;
#11147=EDGE_CURVE ( 'NONE', #21025, #26276, #11837, .T. ) ;
#11149=CARTESIAN_POINT ( 'NONE',  ( -5.622872871577873966, 37.67617187499999432, -13.57481594606304753 ) ) ;
#11154=CARTESIAN_POINT ( 'NONE',  ( -5.622872871577873077, 37.67617187499999432, -13.57481594606304753 ) ) ;
#11155=CARTESIAN_POINT ( 'NONE',  ( 9.295050272127046043, 38.66835937608393436, -9.295050272127046043 ) ) ;
#11157=ORIENTED_EDGE ( 'NONE', *, *, #20458, .T. ) ;
#11167=FACE_OUTER_BOUND ( 'NONE', #1119, .T. ) ;
#11174=ORIENTED_EDGE ( 'NONE', *, *, #6347, .T. ) ;
#11192=CARTESIAN_POINT ( 'NONE',  ( 13.14518615778179900, 35.54296875108394715, 5.444914386472293977 ) ) ;
#11193=CARTESIAN_POINT ( 'NONE',  ( 9.598844408820459861, 36.63437500216787157, 9.598844408820456309 ) ) ;
#11204=EDGE_CURVE ( 'NONE', #17571, #21956, #23504, .T. ) ;
#11208=FILL_AREA_STYLE_COLOUR ( '', #7776 ) ;
#11212=FACE_OUTER_BOUND ( 'NONE', #23422, .T. ) ;
#11213=AXIS2_PLACEMENT_3D ( 'NONE', #26259, #6859, #13252 ) ;
#11215=CARTESIAN_POINT ( 'NONE',  ( 13.14518615778179900, 36.23750000108393010, -5.444914386472297529 ) ) ;
#11219=CARTESIAN_POINT ( 'NONE',  ( -8.312177448680279460E-16, 39.21406249999999716, -13.57481594606304576 ) ) ;
#11244=CARTESIAN_POINT ( 'NONE',  ( 13.14518615778179722, 33.85625000108393579, -5.444914386472297529 ) ) ;
#11253=CARTESIAN_POINT ( 'NONE',  ( 0.000000000000000000, 40.99999999999999289, 0.000000000000000000 ) ) ;
#11263=VERTEX_POINT ( 'NONE', #8252 ) ;
#11287=CARTESIAN_POINT ( 'NONE',  ( -9.295050272127044266, 36.88242187608393152, 9.295050272127047819 ) ) ;
#11292=CARTESIAN_POINT ( 'NONE',  ( -9.295050272127044266, 37.67617187608393436, 9.295050272127047819 ) ) ;
#11293=CARTESIAN_POINT ( 'NONE',  ( -9.598844408820454532, 36.33671874999999574, 9.598844408820459861 ) ) ;
#11299=CARTESIAN_POINT ( 'NONE',  ( -13.57481594606304576, 33.90585937500000568, 5.622872871577880183 ) ) ;
#11300=CARTESIAN_POINT ( 'NONE',  ( -9.295050272127044266, 33.50898437608393010, 9.295050272127047819 ) ) ;
#11311=EDGE_CURVE ( 'NONE', #3364, #34, #25509, .T. ) ;
#11335=CARTESIAN_POINT ( 'NONE',  ( -13.14518615778179544, 36.78320312608393294, 0.000000000000000000 ) ) ;
#11336=CARTESIAN_POINT ( 'NONE',  ( -13.57481594606304576, 37.97382812716787726, 5.622872871577880183 ) ) ;
#11347=CARTESIAN_POINT ( 'NONE',  ( 2.493653234604083739E-15, 31.77265625216787370, 13.57481594606304576 ) ) ;
#11356=CARTESIAN_POINT ( 'NONE',  ( 5.444914386472297529, 35.54296875108393294, -13.14518615778179900 ) ) ;
#11386=ORIENTED_EDGE ( 'NONE', *, *, #17480, .F. ) ;
#11388=CARTESIAN_POINT ( 'NONE',  ( -8.049105076161786076E-16, 33.21132812608393436, -13.14518615778179544 ) ) ;
#11392=AXIS2_PLACEMENT_3D ( 'NONE', #14965, #17256, #21412 ) ;
#11396=CYLINDRICAL_SURFACE ( 'NONE', #6380, 13.57481594606304576 ) ;
#11430=CARTESIAN_POINT ( 'NONE',  ( 9.295050272127047819, 37.08085937608393579, 9.295050272127046043 ) ) ;
#11436=CARTESIAN_POINT ( 'NONE',  ( 5.444914386472302859, 38.61875000108392442, 13.14518615778179189 ) ) ;
#11441=CARTESIAN_POINT ( 'NONE',  ( -5.622872871577873077, 32.11992187499999574, -13.57481594606304753 ) ) ;
#11442=CARTESIAN_POINT ( 'NONE',  ( -13.14518615778179544, 33.40976562608393863, 0.000000000000000000 ) ) ;
#11458=SURFACE_SIDE_STYLE ('',( #15601 ) ) ;
#11478=CARTESIAN_POINT ( 'NONE',  ( -9.295050272127044266, 32.11992187608393579, 9.295050272127047819 ) ) ;
#11479=CARTESIAN_POINT ( 'NONE',  ( -9.598844408820454532, 34.05468750216788010, 9.598844408820459861 ) ) ;
#11499=CARTESIAN_POINT ( 'NONE',  ( 13.14518615778179544, 36.98164062608393010, -1.609821015232357215E-15 ) ) ;
#11516=CARTESIAN_POINT ( 'NONE',  ( 2.493653234604083739E-15, 34.05468749999999289, 13.57481594606304576 ) ) ;
#11526=CARTESIAN_POINT ( 'NONE',  ( 2.414731522848535132E-15, 32.81445312608393294, 13.14518615778179544 ) ) ;
#11569=CARTESIAN_POINT ( 'NONE',  ( -8.049105076161786076E-16, 35.79101562608394005, -13.14518615778179544 ) ) ;
#11574=CARTESIAN_POINT ( 'NONE',  ( 13.14518615778179722, 33.26093750108393721, -5.444914386472297529 ) ) ;
#11581=CARTESIAN_POINT ( 'NONE',  ( -13.57481594606304753, 33.80664062500000000, -5.622872871577873077 ) ) ;
#11582=CARTESIAN_POINT ( 'NONE',  ( 5.444914386472297529, 34.74921875108394431, -13.14518615778179900 ) ) ;
#11611=DIRECTION ( 'NONE',  ( -0.000000000000000000, -1.000000000000000000, -0.000000000000000000 ) ) ;
#11615=CARTESIAN_POINT ( 'NONE',  ( 5.444914386472302859, 34.65000000108393863, 13.14518615778179189 ) ) ;
#11616=CARTESIAN_POINT ( 'NONE',  ( -5.622872871577873077, 34.89804687716787868, 13.57481594606304753 ) ) ;
#11634=LINE ( 'NONE', #695, #15500 ) ;
#11638=CARTESIAN_POINT ( 'NONE',  ( 5.622872871577976994, 40.75195312499999289, -13.57481594606294095 ) ) ;
#11640=CARTESIAN_POINT ( 'NONE',  ( 5.444914386472302859, 33.65781250108393152, 13.14518615778179189 ) ) ;
#11644=CARTESIAN_POINT ( 'NONE',  ( -9.598844408820458085, 35.34453124999998863, -9.598844408820458085 ) ) ;
#11646=DIRECTION ( 'NONE',  ( -0.000000000000000000, -1.000000000000000000, -0.000000000000000000 ) ) ;
#11647=CARTESIAN_POINT ( 'NONE',  ( -5.622872871577920151, 35.39414062716787868, -13.57481594606300135 ) ) ;
#11649=EDGE_LOOP ( 'NONE', ( #23077, #2742, #13361, #9566 ) ) ;
#11655=CARTESIAN_POINT ( 'NONE',  ( -8.312177448680279460E-16, 36.13828125216787157, -13.57481594606304576 ) ) ;
#11671=CARTESIAN_POINT ( 'NONE',  ( -13.14518615778179544, 34.20351562608393436, 0.000000000000000000 ) ) ;
#11686=ORIENTED_EDGE ( 'NONE', *, *, #1447, .T. ) ;
#11692=ORIENTED_EDGE ( 'NONE', *, *, #3251, .F. ) ;
#11711=CARTESIAN_POINT ( 'NONE',  ( -9.295050272127046043, 36.68398437608393436, -9.295050272127046043 ) ) ;
#11717=CARTESIAN_POINT ( 'NONE',  ( -9.295050272127044266, 33.70742187608393436, 9.295050272127047819 ) ) ;
#11723=CARTESIAN_POINT ( 'NONE',  ( -13.57481594606304576, 34.69960937499999432, 5.622872871577880183 ) ) ;
#11724=CARTESIAN_POINT ( 'NONE',  ( -13.14518615778179900, 32.56640625108394005, -5.444914386472297529 ) ) ;
#11729=EDGE_CURVE ( 'NONE', #7953, #8513, #8018, .T. ) ;
#11738=CARTESIAN_POINT ( 'NONE',  ( 9.598844408820456309, 32.07031250216787299, -9.598844408820458085 ) ) ;
#11740=EDGE_CURVE ( 'NONE', #19588, #19872, #6930, .T. ) ;
#11762=CARTESIAN_POINT ( 'NONE',  ( 13.14518615778179900, 34.84843750108393579, -5.444914386472297529 ) ) ;
#11763=CARTESIAN_POINT ( 'NONE',  ( 9.598844408820456309, 32.86406250216787583, -9.598844408820458085 ) ) ;
#11777=EDGE_CURVE ( 'NONE', #28027, #8402, #18603, .T. ) ;
#11785=CARTESIAN_POINT ( 'NONE',  ( 5.444914386472302859, 32.86406250108392868, 13.14518615778179189 ) ) ;
#11798=VERTEX_POINT ( 'NONE', #22884 ) ;
#11816=CARTESIAN_POINT ( 'NONE',  ( -13.14518615778179189, 32.66562500108393863, 5.444914386472304635 ) ) ;
#11824=CARTESIAN_POINT ( 'NONE',  ( 9.598844408820456309, 36.03906250216787299, -9.598844408820458085 ) ) ;
#11835=CARTESIAN_POINT ( 'NONE',  ( 2.493653234604083739E-15, 39.71015625216787015, 13.57481594606304576 ) ) ;
#11837=( BOUNDED_CURVE ( )  B_SPLINE_CURVE ( 2, ( #22684, #3154, #11824, #20401, #27107, #25095, #1171, #11965, #7558 ),
 .UNSPECIFIED., .F., .F. ) 
 B_SPLINE_CURVE_WITH_KNOTS ( ( 3, 2, 2, 2, 3 ),
 ( 0.4375000000000003331, 0.4479166666666669627, 0.4583333333333335369, 0.4687500000000001665, 0.4791666666666667962 ),
 .UNSPECIFIED. ) 
 CURVE ( )  GEOMETRIC_REPRESENTATION_ITEM ( )  RATIONAL_B_SPLINE_CURVE ( ( 0.9999999999999975575, 0.9238795325112891810, 1.000000000000000000, 0.9238795325112867385, 1.000000000000000000, 0.9238795325112867385, 1.000000000000000000, 0.9238795325112859613, 1.000000000000000888 ) ) 
 REPRESENTATION_ITEM ( '' )  );
#11855=CARTESIAN_POINT ( 'NONE',  ( 13.14518615778179544, 36.38632812608393863, -1.609821015232357215E-15 ) ) ;
#11861=CARTESIAN_POINT ( 'NONE',  ( 2.414731522848535132E-15, 33.80664062608393294, 13.14518615778179544 ) ) ;
#11867=CARTESIAN_POINT ( 'NONE',  ( 5.622872871577871301, 33.60820312499998863, -13.57481594606304753 ) ) ;
#11868=CARTESIAN_POINT ( 'NONE',  ( 9.295050272127046043, 34.69960937608393436, -9.295050272127046043 ) ) ;
#11876=CARTESIAN_POINT ( 'NONE',  ( 2.493653234604083739E-15, 34.05468749999999289, 13.57481594606304576 ) ) ;
#11879=CARTESIAN_POINT ( 'NONE',  ( -9.598844408820458085, 34.65000000216787868, -9.598844408820458085 ) ) ;
#11886=DIRECTION ( 'NONE',  ( 0.000000000000000000, 0.000000000000000000, -1.000000000000000000 ) ) ;
#11900=CARTESIAN_POINT ( 'NONE',  ( -5.444914386472297529, 35.04687500108393294, -13.14518615778179900 ) ) ;
#11901=CARTESIAN_POINT ( 'NONE',  ( -5.622872871577873077, 35.39414062716787157, -13.57481594606304753 ) ) ;
#11924=CARTESIAN_POINT ( 'NONE',  ( -5.622872871578010745, 32.91367187499999858, -13.57481594606290898 ) ) ;
#11926=CARTESIAN_POINT ( 'NONE',  ( -13.14518615778179900, 33.36015625108393579, -5.444914386472297529 ) ) ;
#11932=LINE ( 'NONE', #5262, #16223 ) ;
#11939=ADVANCED_FACE ( 'NONE', ( #12570 ), #27718, .F. ) ;
#11949=ORIENTED_EDGE ( 'NONE', *, *, #9027, .F. ) ;
#11951=AXIS2_PLACEMENT_3D ( 'NONE', #6813, #15502, #4840 ) ;
#11965=CARTESIAN_POINT ( 'NONE',  ( 5.622872871577832221, 35.79101562716787299, 13.57481594606309194 ) ) ;
#11983=ORIENTED_EDGE ( 'NONE', *, *, #24799, .F. ) ;
#11999=ORIENTED_EDGE ( 'NONE', *, *, #16443, .T. ) ;
#12000=CARTESIAN_POINT ( 'NONE',  ( 9.295050272127047819, 36.28710937608393294, 9.295050272127046043 ) ) ;
#12022=ORIENTED_EDGE ( 'NONE', *, *, #27964, .F. ) ;
#12028=DIRECTION ( 'NONE',  ( 0.000000000000000000, -0.000000000000000000, 1.000000000000000000 ) ) ;
#12037=CARTESIAN_POINT ( 'NONE',  ( 13.14518615778179544, 32.41757812608393863, -1.609821015232357215E-15 ) ) ;
#12038=CARTESIAN_POINT ( 'NONE',  ( -5.622872871577873077, 33.80664062716786589, -13.57481594606304753 ) ) ;
#12058=ORIENTED_EDGE ( 'NONE', *, *, #10172, .F. ) ;
#12061=CARTESIAN_POINT ( 'NONE',  ( -8.049105076161786076E-16, 32.41757812608393863, -13.14518615778179544 ) ) ;
#12067=ADVANCED_FACE ( 'NONE', ( #6184 ), #1919, .F. ) ;
#12107=EDGE_CURVE ( 'NONE', #10223, #13527, #12901, .T. ) ;
#12121=CARTESIAN_POINT ( 'NONE',  ( -5.444914386472297529, 40.40468750108393436, -13.14518615778179722 ) ) ;
#12128=CARTESIAN_POINT ( 'NONE',  ( -9.295050272127046043, 31.92148437608393508, -9.295050272127046043 ) ) ;
#12137=CARTESIAN_POINT ( 'NONE',  ( -5.444914386472299306, 33.75703125108393721, 13.14518615778179722 ) ) ;
#12143=CARTESIAN_POINT ( 'NONE',  ( 13.14518615778179900, 32.16953125108393152, 5.444914386472293977 ) ) ;
#12173=CARTESIAN_POINT ( 'NONE',  ( -8.312177448680279460E-16, 40.80156249999999574, -13.57481594606304576 ) ) ;
#12174=CARTESIAN_POINT ( 'NONE',  ( -13.14518615778179189, 39.01562500108393294, 5.444914386472304635 ) ) ;
#12191=DIRECTION ( 'NONE',  ( -0.000000000000000000, -1.000000000000000000, -0.000000000000000000 ) ) ;
#12206=CARTESIAN_POINT ( 'NONE',  ( -13.57481594606304753, 40.95039062499999005, -5.622872871577872189 ) ) ;
#12209=ORIENTED_EDGE ( 'NONE', *, *, #14702, .T. ) ;
#12211=CARTESIAN_POINT ( 'NONE',  ( 9.295050272127047819, 40.25585937608393294, 9.295050272127046043 ) ) ;
#12212=CARTESIAN_POINT ( 'NONE',  ( -9.598844408820458085, 39.41250000216787441, -9.598844408820458085 ) ) ;
#12219=ORIENTED_EDGE ( 'NONE', *, *, #27950, .T. ) ;
#12254=ORIENTED_EDGE ( 'NONE', *, *, #8613, .F. ) ;
#12268=CARTESIAN_POINT ( 'NONE',  ( 5.444914386472297529, 33.36015625108393579, -13.14518615778179900 ) ) ;
#12275=CARTESIAN_POINT ( 'NONE',  ( -5.444914386472297529, 31.87187500108393223, -13.14518615778179722 ) ) ;
#12284=CARTESIAN_POINT ( 'NONE',  ( 9.295050272127046043, 32.31835937608393294, -9.295050272127046043 ) ) ;
#12288=CARTESIAN_POINT ( 'NONE',  ( 5.622872871577961895, 35.19570312499999432, -13.57481594606295339 ) ) ;
#12307=CARTESIAN_POINT ( 'NONE',  ( 9.295050272127046043, 40.45429687608393721, -9.295050272127046043 ) ) ;
#12317=CARTESIAN_POINT ( 'NONE',  ( -13.57481594606304753, 38.56914062500000284, -5.622872871577873077 ) ) ;
#12318=CARTESIAN_POINT ( 'NONE',  ( 13.14518615778179900, 39.31328125108392868, 5.444914386472293977 ) ) ;
#12351=CARTESIAN_POINT ( 'NONE',  ( -8.312177448680279460E-16, 39.21406249999999716, -13.57481594606304576 ) ) ;
#12355=ORIENTED_EDGE ( 'NONE', *, *, #16469, .T. ) ;
#12357=CARTESIAN_POINT ( 'NONE',  ( -5.444914386472297529, 39.80937500108392868, -13.14518615778179900 ) ) ;
#12384=CARTESIAN_POINT ( 'NONE',  ( 9.598844408820459861, 39.71015624999999716, 9.598844408820456309 ) ) ;
#12397=CARTESIAN_POINT ( 'NONE',  ( -5.444914386472299306, 39.11484375108393863, 13.14518615778179722 ) ) ;
#12401=EDGE_LOOP ( 'NONE', ( #1046, #17570, #21566, #26277, #10144, #22144, #4984, #16525 ) ) ;
#12403=CARTESIAN_POINT ( 'NONE',  ( 2.493653234604083739E-15, 34.15390625216787157, 13.57481594606304576 ) ) ;
#12408=CARTESIAN_POINT ( 'NONE',  ( 9.295050272127047819, 33.11210937608393579, 9.295050272127046043 ) ) ;
#12423=VERTEX_POINT ( 'NONE', #12403 ) ;
#12425=CARTESIAN_POINT ( 'NONE',  ( 5.622872871577924592, 32.61601562716786873, 13.57481594606299957 ) ) ;
#12427=ORIENTED_EDGE ( 'NONE', *, *, #3913, .T. ) ;
#12434=ORIENTED_EDGE ( 'NONE', *, *, #17480, .T. ) ;
#12447=CARTESIAN_POINT ( 'NONE',  ( 9.598844408820459861, 39.71015624999999716, 9.598844408820456309 ) ) ;
#12448=CARTESIAN_POINT ( 'NONE',  ( -8.312177448680279460E-16, 31.37578125216787583, -13.57481594606304576 ) ) ;
#12453=EDGE_CURVE ( 'NONE', #26359, #6320, #26430, .T. ) ;
#12469=CARTESIAN_POINT ( 'NONE',  ( -5.622872871577688336, 32.21914062716787441, -13.57481594606323050 ) ) ;
#12487=CARTESIAN_POINT ( 'NONE',  ( 9.295050272127046043, 38.86679687608393863, -9.295050272127046043 ) ) ;
#12489=DIRECTION ( 'NONE',  ( 0.000000000000000000, -1.000000000000000000, 0.000000000000000000 ) ) ;
#12504=CARTESIAN_POINT ( 'NONE',  ( 9.295050272127046043, 40.25585937608393294, -9.295050272127046043 ) ) ;
#12507=CARTESIAN_POINT ( 'NONE',  ( 13.57481594606304931, 35.79101562499999289, 5.622872871577868636 ) ) ;
#12523=EDGE_LOOP ( 'NONE', ( #3753, #5091, #8553, #9757 ) ) ;
#12543=CARTESIAN_POINT ( 'NONE',  ( -13.14518615778179900, 32.76484375108393010, -5.444914386472297529 ) ) ;
#12567=ADVANCED_FACE ( 'NONE', ( #12686 ), #21546, .F. ) ;
#12570=FACE_OUTER_BOUND ( 'NONE', #16407, .T. ) ;
#12574=CARTESIAN_POINT ( 'NONE',  ( 13.14518615778179544, 34.60039062608392868, -1.609821015232357215E-15 ) ) ;
#12580=FACE_OUTER_BOUND ( 'NONE', #11087, .T. ) ;
#12588=CARTESIAN_POINT ( 'NONE',  ( 2.493653234604083739E-15, 40.40468749999999432, 13.57481594606304576 ) ) ;
#12589=CARTESIAN_POINT ( 'NONE',  ( 13.14518615778179900, 39.41250000108393436, -5.444914386472297529 ) ) ;
#12595=ADVANCED_FACE ( 'NONE', ( #2164 ), #13093, .F. ) ;
#12618=CYLINDRICAL_SURFACE ( 'NONE', #1310, 13.57481594606304576 ) ;
#12643=CARTESIAN_POINT ( 'NONE',  ( -9.598844408820454532, 38.71796874999999716, 9.598844408820459861 ) ) ;
#12651=CARTESIAN_POINT ( 'NONE',  ( 13.14518615778179900, 38.61875000108393152, -5.444914386472297529 ) ) ;
#12673=CARTESIAN_POINT ( 'NONE',  ( -5.622872871577873966, 33.01289062716787726, -13.57481594606304753 ) ) ;
#12679=CARTESIAN_POINT ( 'NONE',  ( 2.414731522848535132E-15, 38.37070312608393152, 13.14518615778179544 ) ) ;
#12686=FACE_OUTER_BOUND ( 'NONE', #15970, .T. ) ;
#12713=CIRCLE ( 'NONE', #20025, 15.57481594606304576 ) ;
#12719=CARTESIAN_POINT ( 'NONE',  ( 13.14518615778179900, 40.30546875108393579, 5.444914386472293977 ) ) ;
#12725=CARTESIAN_POINT ( 'NONE',  ( 5.444914386472297529, 40.50390625108394005, -13.14518615778179722 ) ) ;
#12728=CARTESIAN_POINT ( 'NONE',  ( -5.622872871577965448, 37.97382812499999716, 13.57481594606295161 ) ) ;
#12732=CARTESIAN_POINT ( 'NONE',  ( 13.57481594606304753, 40.65273437499998721, -5.622872871577873077 ) ) ;
#12733=CARTESIAN_POINT ( 'NONE',  ( 13.14518615778179900, 40.10703125108393152, 5.444914386472293977 ) ) ;
#12750=CARTESIAN_POINT ( 'NONE',  ( -13.57481594606304398, 37.08085937499999574, 5.622872871577880183 ) ) ;
#12766=CARTESIAN_POINT ( 'NONE',  ( 5.622872871577870413, 33.60820312499999574, -13.57481594606304753 ) ) ;
#12770=DIRECTION ( 'NONE',  ( 0.000000000000000000, 0.000000000000000000, 1.000000000000000000 ) ) ;
#12772=CARTESIAN_POINT ( 'NONE',  ( -13.14518615778179189, 39.21406250108392300, 5.444914386472304635 ) ) ;
#12790=CARTESIAN_POINT ( 'NONE',  ( -8.049105076161786076E-16, 38.76757812608393294, -13.14518615778179544 ) ) ;
#12804=ADVANCED_FACE ( 'NONE', ( #20249 ), #11396, .F. ) ;
#12814=CARTESIAN_POINT ( 'NONE',  ( -5.444914386472299306, 36.73359375108393010, 13.14518615778179722 ) ) ;
#12834=CARTESIAN_POINT ( 'NONE',  ( 5.444914386472302859, 32.26875000108393721, 13.14518615778179189 ) ) ;
#12835=CARTESIAN_POINT ( 'NONE',  ( -13.14518615778179544, 40.55351562608393579, 0.000000000000000000 ) ) ;
#12853=CARTESIAN_POINT ( 'NONE',  ( -5.444914386472297529, 40.60312500108393863, -13.14518615778179900 ) ) ;
#12864=CARTESIAN_POINT ( 'NONE',  ( 13.57481594606304931, 35.79101562499999289, 5.622872871577869525 ) ) ;
#12865=CARTESIAN_POINT ( 'NONE',  ( 5.444914386472297529, 38.71796875108393721, -13.14518615778179900 ) ) ;
#12873=CARTESIAN_POINT ( 'NONE',  ( -13.57481594606304576, 38.71796875216787726, 0.000000000000000000 ) ) ;
#12880=CARTESIAN_POINT ( 'NONE',  ( -13.57481594606304576, 36.33671875216787583, 0.000000000000000000 ) ) ;
#12889=LINE ( 'NONE', #26169, #26315 ) ;
#12894=ORIENTED_EDGE ( 'NONE', *, *, #11311, .T. ) ;
#12895=CARTESIAN_POINT ( 'NONE',  ( -13.57481594606304576, 39.41249999999999432, 0.000000000000000000 ) ) ;
#12901=( BOUNDED_CURVE ( )  B_SPLINE_CURVE ( 2, ( #17286, #17143, #21999, #10859, #2475, #6734, #25844, #23712, #19151 ),
 .UNSPECIFIED., .F., .F. ) 
 B_SPLINE_CURVE_WITH_KNOTS ( ( 3, 2, 2, 2, 3 ),
 ( 0.3541666666666666852, 0.3645833333333332593, 0.3749999999999998890, 0.3854166666666665741, 0.3958333333333331483 ),
 .UNSPECIFIED. ) 
 CURVE ( )  GEOMETRIC_REPRESENTATION_ITEM ( )  RATIONAL_B_SPLINE_CURVE ( ( 1.000000000000000000, 0.9238795325112867385, 1.000000000000000000, 0.9238795325112867385, 1.000000000000000000, 0.9238795325112867385, 1.000000000000000000, 0.9238795325112879597, 0.9999999999999987788 ) ) 
 REPRESENTATION_ITEM ( '' )  );
#12902=CARTESIAN_POINT ( 'NONE',  ( 13.14518615778179900, 36.43593750108392726, -5.444914386472297529 ) ) ;
#12903=CARTESIAN_POINT ( 'NONE',  ( -13.57481594606304576, 36.33671875216787583, 0.000000000000000000 ) ) ;
#12912=CARTESIAN_POINT ( 'NONE',  ( -13.57481594606304576, 33.95546875216787441, 0.000000000000000000 ) ) ;
#12947=ADVANCED_FACE ( 'NONE', ( #3844 ), #6032, .F. ) ;
#12948=CARTESIAN_POINT ( 'NONE',  ( 9.295050272127047819, 36.08867187608392868, 9.295050272127046043 ) ) ;
#12964=CARTESIAN_POINT ( 'NONE',  ( 0.000000000000000000, 40.99999999999999289, 0.000000000000000000 ) ) ;
#12984=EDGE_CURVE ( 'NONE', #21530, #7430, #2315, .T. ) ;
#12987=ORIENTED_EDGE ( 'NONE', *, *, #7591, .F. ) ;
#12989=CARTESIAN_POINT ( 'NONE',  ( -5.444914386472299306, 39.31328125108394289, 13.14518615778179722 ) ) ;
#12994=CARTESIAN_POINT ( 'NONE',  ( -13.14518615778179544, 39.16445312608393436, 0.000000000000000000 ) ) ;
#13001=CARTESIAN_POINT ( 'NONE',  ( 13.57481594606304753, 36.68398437499999432, -5.622872871577873077 ) ) ;
#13002=CARTESIAN_POINT ( 'NONE',  ( 13.14518615778179900, 36.23750000108393010, -5.444914386472297529 ) ) ;
#13012=CARTESIAN_POINT ( 'NONE',  ( -5.622872871577816234, 38.56914062716787583, -13.57481594606310260 ) ) ;
#13017=CARTESIAN_POINT ( 'NONE',  ( 2.493653234604083739E-15, 34.84843749999999574, 13.57481594606304576 ) ) ;
#13041=CARTESIAN_POINT ( 'NONE',  ( 2.414731522848535132E-15, 35.39414062608393863, 13.14518615778179544 ) ) ;
#13042=CARTESIAN_POINT ( 'NONE',  ( 5.622872871577878406, 38.17226562716786731, 13.57481594606304576 ) ) ;
#13059=CARTESIAN_POINT ( 'NONE',  ( -5.444914386472297529, 40.40468750108393436, -13.14518615778179900 ) ) ;
#13062=CARTESIAN_POINT ( 'NONE',  ( 9.598844408820459861, 38.91640624999999432, 9.598844408820456309 ) ) ;
#13087=CARTESIAN_POINT ( 'NONE',  ( -13.14518615778179722, 37.32890625108393579, -5.444914386472297529 ) ) ;
#13093=CYLINDRICAL_SURFACE ( 'NONE', #8678, 13.57481594606304576 ) ;
#13094=AXIS2_PLACEMENT_3D ( 'NONE', #6509, #15185, #12770 ) ;
#13102=DIRECTION ( 'NONE',  ( -0.000000000000000000, -1.000000000000000000, -0.000000000000000000 ) ) ;
#13111=EDGE_CURVE ( 'NONE', #8015, #15078, #6262, .T. ) ;
#13133=CARTESIAN_POINT ( 'NONE',  ( 9.295050272127046043, 39.66054687608393436, -9.295050272127046043 ) ) ;
#13138=CARTESIAN_POINT ( 'NONE',  ( 2.414731522848535132E-15, 36.98164062608393721, 13.14518615778179544 ) ) ;
#13140=CARTESIAN_POINT ( 'NONE',  ( -9.598844408820454532, 37.92421874999999432, 9.598844408820459861 ) ) ;
#13146=CARTESIAN_POINT ( 'NONE',  ( -5.622872871577873077, 37.18007812500000853, 13.57481594606304753 ) ) ;
#13147=CARTESIAN_POINT ( 'NONE',  ( -13.14518615778179189, 36.63437500108393152, 5.444914386472304635 ) ) ;
#13151=EDGE_CURVE ( 'NONE', #26276, #3364, #17496, .T. ) ;
#13159=LINE ( 'NONE', #4784, #24938 ) ;
#13170=CARTESIAN_POINT ( 'NONE',  ( 9.598844408820456309, 32.76484374999999716, -9.598844408820458085 ) ) ;
#13175=CARTESIAN_POINT ( 'NONE',  ( 2.493653234604083739E-15, 36.43593749999999432, 13.57481594606304576 ) ) ;
#13182=CARTESIAN_POINT ( 'NONE',  ( -9.295050272127046043, 36.68398437608393436, -9.295050272127046043 ) ) ;
#13183=CARTESIAN_POINT ( 'NONE',  ( 13.57481594606304576, 38.32109375216786873, -1.662435489736055892E-15 ) ) ;
#13188=ORIENTED_EDGE ( 'NONE', *, *, #27304, .T. ) ;
#13195=DIRECTION ( 'NONE',  ( -0.000000000000000000, -1.000000000000000000, -0.000000000000000000 ) ) ;
#13205=CARTESIAN_POINT ( 'NONE',  ( 5.444914386472302859, 35.24531250108393010, 13.14518615778179189 ) ) ;
#13224=ORIENTED_EDGE ( 'NONE', *, *, #10156, .F. ) ;
#13227=ORIENTED_EDGE ( 'NONE', *, *, #27428, .F. ) ;
#13231=CARTESIAN_POINT ( 'NONE',  ( 9.295050272127046043, 34.69960937608393436, -9.295050272127046043 ) ) ;
#13252=DIRECTION ( 'NONE',  ( 0.000000000000000000, 0.000000000000000000, -1.000000000000000000 ) ) ;
#13265=( BOUNDED_CURVE ( )  B_SPLINE_CURVE ( 2, ( #13017, #1809, #2231, #21755, #28163, #25734, #2372, #19465, #11030 ),
 .UNSPECIFIED., .F., .F. ) 
 B_SPLINE_CURVE_WITH_KNOTS ( ( 3, 2, 2, 2, 3 ),
 ( 0.6458333333333333703, 0.6562500000000000000, 0.6666666666666665186, 0.6770833333333332593, 0.6874999999999997780 ),
 .UNSPECIFIED. ) 
 CURVE ( )  GEOMETRIC_REPRESENTATION_ITEM ( )  RATIONAL_B_SPLINE_CURVE ( ( 1.000000000000000000, 0.9238795325112867385, 1.000000000000000000, 0.9238795325112867385, 1.000000000000000000, 0.9238795325112867385, 1.000000000000000000, 0.9238795325112884038, 0.9999999999999983347 ) ) 
 REPRESENTATION_ITEM ( '' )  );
#13273=CARTESIAN_POINT ( 'NONE',  ( -8.049105076161786076E-16, 38.96601562608393721, -13.14518615778179544 ) ) ;
#13279=CARTESIAN_POINT ( 'NONE',  ( -13.14518615778179722, 37.52734375108393294, -5.444914386472297529 ) ) ;
#13287=CARTESIAN_POINT ( 'NONE',  ( -8.312177448680279460E-16, 37.62656249999999858, -13.57481594606304576 ) ) ;
#13288=CARTESIAN_POINT ( 'NONE',  ( 13.14518615778179900, 38.51953125108393294, 5.444914386472293977 ) ) ;
#13322=CARTESIAN_POINT ( 'NONE',  ( -5.622872871577816234, 39.26367187500000000, -13.57481594606310260 ) ) ;
#13327=EDGE_CURVE ( 'NONE', #17637, #5570, #8086, .T. ) ;
#13330=CARTESIAN_POINT ( 'NONE',  ( -5.444914386472299306, 37.72578125108395142, 13.14518615778179722 ) ) ;
#13331=CARTESIAN_POINT ( 'NONE',  ( 9.598844408820459861, 35.84062500216786873, 9.598844408820456309 ) ) ;
#13347=CYLINDRICAL_SURFACE ( 'NONE', #8891, 13.57481594606304576 ) ;
#13349=CARTESIAN_POINT ( 'NONE',  ( -13.14518615778179189, 35.04687500108393294, 5.444914386472304635 ) ) ;
#13356=CARTESIAN_POINT ( 'NONE',  ( -8.312177448680279460E-16, 35.34453125216787583, -13.57481594606304576 ) ) ;
#13361=ORIENTED_EDGE ( 'NONE', *, *, #7016, .T. ) ;
#13372=ORIENTED_EDGE ( 'NONE', *, *, #28182, .T. ) ;
#13377=CARTESIAN_POINT ( 'NONE',  ( -13.14518615778179722, 35.74140625108393721, -5.444914386472297529 ) ) ;
#13380=EDGE_LOOP ( 'NONE', ( #12058, #25150, #1968 ) ) ;
#13395=ORIENTED_EDGE ( 'NONE', *, *, #14163, .T. ) ;
#13401=ORIENTED_EDGE ( 'NONE', *, *, #23321, .F. ) ;
#13417=EDGE_LOOP ( 'NONE', ( #27813, #7290, #20410, #25653 ) ) ;
#13419=CARTESIAN_POINT ( 'NONE',  ( 9.295050272127047819, 36.28710937608393294, 9.295050272127046043 ) ) ;
#13425=CARTESIAN_POINT ( 'NONE',  ( -8.049105076161786076E-16, 36.58476562608393579, -13.14518615778179544 ) ) ;
#13431=CARTESIAN_POINT ( 'NONE',  ( 13.57481594606304753, 35.09648437499998863, -5.622872871577873077 ) ) ;
#13432=CARTESIAN_POINT ( 'NONE',  ( 5.444914386472302859, 36.83281250108392868, 13.14518615778179189 ) ) ;
#13442=( BOUNDED_CURVE ( )  B_SPLINE_CURVE ( 2, ( #27415, #9873, #16429, #27696, #5895, #7740, #10136, #5754, #7878 ),
 .UNSPECIFIED., .F., .F. ) 
 B_SPLINE_CURVE_WITH_KNOTS ( ( 3, 2, 2, 2, 3 ),
 ( 0.1041666666666664909, 0.1145833333333332732, 0.1250000000000000833, 0.1354166666666668517, 0.1458333333333336757 ),
 .UNSPECIFIED. ) 
 CURVE ( )  GEOMETRIC_REPRESENTATION_ITEM ( )  RATIONAL_B_SPLINE_CURVE ( ( 1.000000000000001332, 0.9238795325112854062, 1.000000000000000000, 0.9238795325112867385, 1.000000000000000000, 0.9238795325112867385, 1.000000000000000000, 0.9238795325112842960, 1.000000000000002442 ) ) 
 REPRESENTATION_ITEM ( '' )  );
#13469=CARTESIAN_POINT ( 'NONE',  ( -5.444914386472297529, 38.22187500108393010, -13.14518615778179900 ) ) ;
#13470=CARTESIAN_POINT ( 'NONE',  ( -9.598844408820454532, 38.81718750216787583, 9.598844408820459861 ) ) ;
#13490=( BOUNDED_CURVE ( )  B_SPLINE_CURVE ( 2, ( #11876, #16731, #25430, #27167, #8175, #16447, #21018, #1225, #9889 ),
 .UNSPECIFIED., .F., .T. ) 
 B_SPLINE_CURVE_WITH_KNOTS ( ( 3, 2, 2, 2, 3 ),
 ( 0.7291666666666668517, 0.7395833333333334814, 0.7500000000000001110, 0.7604166666666667407, 0.7708333333333333703 ),
 .UNSPECIFIED. ) 
 CURVE ( )  GEOMETRIC_REPRESENTATION_ITEM ( )  RATIONAL_B_SPLINE_CURVE ( ( 0.9999999999999983347, 0.9238795325112884038, 1.000000000000000000, 0.9238795325112867385, 1.000000000000000000, 0.9238795325112867385, 1.000000000000000000, 0.9238795325112867385, 1.000000000000000000 ) ) 
 REPRESENTATION_ITEM ( '' )  );
#13497=CARTESIAN_POINT ( 'NONE',  ( 13.14518615778179544, 36.18789062608393436, -1.609821015232357215E-15 ) ) ;
#13527=VERTEX_POINT ( 'NONE', #21769 ) ;
#13528=CARTESIAN_POINT ( 'NONE',  ( -5.444914386472299306, 34.35234375108392868, 13.14518615778179722 ) ) ;
#13534=( BOUNDED_CURVE ( )  B_SPLINE_CURVE ( 2, ( #26524, #24096, #9126, #20394, #4572, #26383, #7262, #17533, #19818 ),
 .UNSPECIFIED., .F., .F. ) 
 B_SPLINE_CURVE_WITH_KNOTS ( ( 3, 2, 2, 2, 3 ),
 ( 0.3541666666666666852, 0.3645833333333332593, 0.3749999999999998890, 0.3854166666666665741, 0.3958333333333331483 ),
 .UNSPECIFIED. ) 
 CURVE ( )  GEOMETRIC_REPRESENTATION_ITEM ( )  RATIONAL_B_SPLINE_CURVE ( ( 1.000000000000000000, 0.9238795325112867385, 1.000000000000000000, 0.9238795325112867385, 1.000000000000000000, 0.9238795325112867385, 1.000000000000000000, 0.9238795325112879597, 0.9999999999999987788 ) ) 
 REPRESENTATION_ITEM ( '' )  );
#13567=CARTESIAN_POINT ( 'NONE',  ( 13.14518615778179900, 36.43593750108392726, -5.444914386472297529 ) ) ;
#13572=ORIENTED_EDGE ( 'NONE', *, *, #21514, .F. ) ;
#13573=CARTESIAN_POINT ( 'NONE',  ( 13.14518615778179544, 37.18007812608393436, -1.609821015232357215E-15 ) ) ;
#13574=CARTESIAN_POINT ( 'NONE',  ( -9.598844408820458085, 36.13828124999999147, -9.598844408820458085 ) ) ;
#13579=CARTESIAN_POINT ( 'NONE',  ( 9.598844408820456309, 32.76484374999999716, -9.598844408820458085 ) ) ;
#13580=CARTESIAN_POINT ( 'NONE',  ( -13.14518615778179189, 35.04687500108393294, 5.444914386472304635 ) ) ;
#13590=CARTESIAN_POINT ( 'NONE',  ( 6.944426393311537993, 31.75150625057403175, -11.16113171639042356 ) ) ;
#13594=CARTESIAN_POINT ( 'NONE',  ( 9.598844408820459861, 36.53515624999999289, 9.598844408820456309 ) ) ;
#13616=CARTESIAN_POINT ( 'NONE',  ( 13.14518615778179900, 32.36796875108393579, 5.444914386472293977 ) ) ;
#13617=CARTESIAN_POINT ( 'NONE',  ( 13.57481594606304576, 33.55859375216787299, -1.662435489736055892E-15 ) ) ;
#13625=VECTOR ( 'NONE', #862, 1000.000000000000000 ) ;
#13641=CARTESIAN_POINT ( 'NONE',  ( 13.14518615778179900, 35.44375000108393436, -5.444914386472297529 ) ) ;
#13651=DIRECTION ( 'NONE',  ( -0.000000000000000000, -1.000000000000000000, -0.000000000000000000 ) ) ;
#13660=EDGE_CURVE ( 'NONE', #6320, #26359, #17750, .T. ) ;
#13670=CARTESIAN_POINT ( 'NONE',  ( -5.444914386472297529, 31.67343750108393863, -13.14518615778179722 ) ) ;
#13710=CARTESIAN_POINT ( 'NONE',  ( -13.14518615778179900, 35.93984375108393436, -5.444914386472297529 ) ) ;
#13716=CARTESIAN_POINT ( 'NONE',  ( -5.444914386472299306, 35.34453125108393579, 13.14518615778179722 ) ) ;
#13722=CARTESIAN_POINT ( 'NONE',  ( 7.171391216998965312, 31.99955315621561525, -11.52591757658528948 ) ) ;
#13723=CARTESIAN_POINT ( 'NONE',  ( 9.295050272127047819, 32.91367187608393152, 9.295050272127046043 ) ) ;
#13728=VERTEX_POINT ( 'NONE', #14178 ) ;
#13755=CARTESIAN_POINT ( 'NONE',  ( -13.14518615778179189, 32.86406250108393579, 5.444914386472304635 ) ) ;
#13756=CARTESIAN_POINT ( 'NONE',  ( -13.57481594606304753, 33.11210937716786873, -5.622872871577873077 ) ) ;
#13772=DIRECTION ( 'NONE',  ( -0.000000000000000000, -1.000000000000000000, -0.000000000000000000 ) ) ;
#13778=CARTESIAN_POINT ( 'NONE',  ( 5.444914386472302859, 37.62656250108393863, 13.14518615778179189 ) ) ;
#13787=ORIENTED_EDGE ( 'NONE', *, *, #22894, .F. ) ;
#13808=CARTESIAN_POINT ( 'NONE',  ( -5.444914386472299306, 32.76484375108393010, 13.14518615778179722 ) ) ;
#13824=ORIENTED_EDGE ( 'NONE', *, *, #21691, .F. ) ;
#13849=CARTESIAN_POINT ( 'NONE',  ( 9.295050272127047819, 34.69960937608393436, 9.295050272127046043 ) ) ;
#13855=CARTESIAN_POINT ( 'NONE',  ( 13.14518615778179722, 34.74921875108395142, 5.444914386472293977 ) ) ;
#13863=CARTESIAN_POINT ( 'NONE',  ( -8.312177448680279460E-16, 32.07031249999999289, -13.57481594606304576 ) ) ;
#13864=CARTESIAN_POINT ( 'NONE',  ( -9.295050272127044266, 32.71523437608393436, 9.295050272127047819 ) ) ;
#13899=CARTESIAN_POINT ( 'NONE',  ( 9.295050272127046043, 34.89804687608393863, -9.295050272127046043 ) ) ;
#13900=CARTESIAN_POINT ( 'NONE',  ( 5.622872871577871301, 32.91367187716787157, -13.57481594606304753 ) ) ;
#13912=CARTESIAN_POINT ( 'NONE',  ( -5.622872871577873966, 31.42539062716787157, -13.57481594606304753 ) ) ;
#13920=CARTESIAN_POINT ( 'NONE',  ( 13.14518615778179900, 32.16953125108393152, 5.444914386472293977 ) ) ;
#13934=CARTESIAN_POINT ( 'NONE',  ( 0.000000000000000000, 40.99999999999999289, -13.57481594606304576 ) ) ;
#13950=CARTESIAN_POINT ( 'NONE',  ( -9.295050272127044266, 34.30273437608393294, 9.295050272127047819 ) ) ;
#13969=CARTESIAN_POINT ( 'NONE',  ( 5.622872871577863307, 39.75976562716787299, 13.57481594606306174 ) ) ;
#13991=CARTESIAN_POINT ( 'NONE',  ( -13.14518615778179900, 37.52734375108393294, -5.444914386472297529 ) ) ;
#14000=CARTESIAN_POINT ( 'NONE',  ( 13.14518615778179722, 36.33671875108393579, 5.444914386472293977 ) ) ;
#14006=CARTESIAN_POINT ( 'NONE',  ( -13.57481594606304753, 33.01289062500000426, -5.622872871577873077 ) ) ;
#14007=CARTESIAN_POINT ( 'NONE',  ( -5.444914386472299306, 35.14609375108393152, 13.14518615778179722 ) ) ;
#14014=ORIENTED_EDGE ( 'NONE', *, *, #20419, .F. ) ;
#14046=CARTESIAN_POINT ( 'NONE',  ( 2.414731522848535132E-15, 33.01289062608393721, 13.14518615778179544 ) ) ;
#14047=CARTESIAN_POINT ( 'NONE',  ( -13.57481594606304576, 34.00507812716787015, 5.622872871577880183 ) ) ;
#14067=CARTESIAN_POINT ( 'NONE',  ( -9.598844408820458085, 32.96328124999999432, -9.598844408820458085 ) ) ;
#14069=CARTESIAN_POINT ( 'NONE',  ( -9.295050272127044266, 33.50898437608393010, 9.295050272127047819 ) ) ;
#14098=CARTESIAN_POINT ( 'NONE',  ( -9.295050272127046043, 34.10429687608393579, -9.295050272127046043 ) ) ;
#14114=ORIENTED_EDGE ( 'NONE', *, *, #15237, .F. ) ;
#14135=CARTESIAN_POINT ( 'NONE',  ( 13.57481594606304931, 38.27148437716787299, 5.622872871577868636 ) ) ;
#14144=CARTESIAN_POINT ( 'NONE',  ( 2.414731522848535132E-15, 34.60039062608393579, 13.14518615778179544 ) ) ;
#14150=CARTESIAN_POINT ( 'NONE',  ( -13.57481594606304576, 34.64999999999999147, 0.000000000000000000 ) ) ;
#14151=CARTESIAN_POINT ( 'NONE',  ( 13.14518615778179900, 33.75703125108393010, 5.444914386472293977 ) ) ;
#14163=EDGE_CURVE ( 'NONE', #10337, #5311, #26256, .T. ) ;
#14178=CARTESIAN_POINT ( 'NONE',  ( -8.312177448680279460E-16, 40.10703125216787157, -13.57481594606304576 ) ) ;
#14182=ORIENTED_EDGE ( 'NONE', *, *, #22553, .T. ) ;
#14185=CARTESIAN_POINT ( 'NONE',  ( -8.049105076161786076E-16, 33.40976562608393863, -13.14518615778179544 ) ) ;
#14186=CARTESIAN_POINT ( 'NONE',  ( 9.598844408820459861, 34.25312500216787015, 9.598844408820456309 ) ) ;
#14207=( BOUNDED_CURVE ( )  B_SPLINE_CURVE ( 2, ( #717, #6968, #143, #17378, #11092, #2291, #2847, #15663, #11516 ),
 .UNSPECIFIED., .F., .F. ) 
 B_SPLINE_CURVE_WITH_KNOTS ( ( 3, 2, 2, 2, 3 ),
 ( 0.6874999999999997780, 0.6979166666666665186, 0.7083333333333333703, 0.7187500000000001110, 0.7291666666666668517 ),
 .UNSPECIFIED. ) 
 CURVE ( )  GEOMETRIC_REPRESENTATION_ITEM ( )  RATIONAL_B_SPLINE_CURVE ( ( 1.000000000000001554, 0.9238795325112850731, 1.000000000000000000, 0.9238795325112867385, 1.000000000000000000, 0.9238795325112867385, 1.000000000000000000, 0.9238795325112850731, 1.000000000000001554 ) ) 
 REPRESENTATION_ITEM ( '' )  );
#14209=CARTESIAN_POINT ( 'NONE',  ( 5.444914386472302859, 32.07031250108393294, 13.14518615778179189 ) ) ;
#14219=CARTESIAN_POINT ( 'NONE',  ( 0.000000000000000000, 40.99999999999999289, 0.000000000000000000 ) ) ;
#14232=VECTOR ( 'NONE', #2250, 1000.000000000000000 ) ;
#14252=CARTESIAN_POINT ( 'NONE',  ( -8.312177448680279460E-16, 40.00781250000000000, -13.57481594606304576 ) ) ;
#14255=AXIS2_PLACEMENT_3D ( 'NONE', #6308, #27090, #7541 ) ;
#14268=CARTESIAN_POINT ( 'NONE',  ( -13.14518615778179722, 40.50390625108394005, -5.444914386472297529 ) ) ;
#14275=CARTESIAN_POINT ( 'NONE',  ( 5.444914386472297529, 32.56640625108394005, -13.14518615778179900 ) ) ;
#14282=CARTESIAN_POINT ( 'NONE',  ( 13.14518615778179544, 34.79882812608394005, -1.609821015232357215E-15 ) ) ;
#14287=CARTESIAN_POINT ( 'NONE',  ( 0.000000000000000000, 40.99999999999999289, 0.000000000000000000 ) ) ;
#14290=CARTESIAN_POINT ( 'NONE',  ( 9.295050272127047819, 32.11992187608393579, 9.295050272127046043 ) ) ;
#14294=LINE ( 'NONE', #16306, #3238 ) ;
#14317=VERTEX_POINT ( 'NONE', #4742 ) ;
#14320=CARTESIAN_POINT ( 'NONE',  ( -9.598844408820458085, 38.51953124999999289, -9.598844408820458085 ) ) ;
#14321=CARTESIAN_POINT ( 'NONE',  ( -9.598844408820458085, 31.47500000216787441, -9.598844408820458085 ) ) ;
#14326=ORIENTED_EDGE ( 'NONE', *, *, #10987, .T. ) ;
#14330=CARTESIAN_POINT ( 'NONE',  ( 2.493653234604083739E-15, 35.64218749999999147, 13.57481594606304576 ) ) ;
#14357=CARTESIAN_POINT ( 'NONE',  ( 13.57481594606304753, 33.50898437499999716, -5.622872871577873966 ) ) ;
#14387=DIRECTION ( 'NONE',  ( 1.000000000000000000, 0.000000000000000000, 0.000000000000000000 ) ) ;
#14409=CARTESIAN_POINT ( 'NONE',  ( -13.14518615778179544, 38.17226562608393436, 0.000000000000000000 ) ) ;
#14416=( BOUNDED_CURVE ( )  B_SPLINE_CURVE ( 2, ( #407, #15343, #21931, #8527, #2548, #15199, #22209, #17212, #6657 ),
 .UNSPECIFIED., .F., .F. ) 
 B_SPLINE_CURVE_WITH_KNOTS ( ( 3, 2, 2, 2, 3 ),
 ( 0.6041666666666668517, 0.6145833333333334814, 0.6250000000000001110, 0.6354166666666667407, 0.6458333333333333703 ),
 .UNSPECIFIED. ) 
 CURVE ( )  GEOMETRIC_REPRESENTATION_ITEM ( )  RATIONAL_B_SPLINE_CURVE ( ( 0.9999999999999983347, 0.9238795325112884038, 1.000000000000000000, 0.9238795325112867385, 1.000000000000000000, 0.9238795325112867385, 1.000000000000000000, 0.9238795325112867385, 1.000000000000000000 ) ) 
 REPRESENTATION_ITEM ( '' )  );
#14417=CARTESIAN_POINT ( 'NONE',  ( -5.444914386472297529, 32.66562500108393863, -13.14518615778179900 ) ) ;
#14424=ORIENTED_EDGE ( 'NONE', *, *, #18554, .T. ) ;
#14431=CARTESIAN_POINT ( 'NONE',  ( -9.295050272127044266, 31.92148437608393508, 9.295050272127047819 ) ) ;
#14434=CARTESIAN_POINT ( 'NONE',  ( 13.57481594606304576, 32.76484375216787015, -1.662435489736055892E-15 ) ) ;
#14444=CARTESIAN_POINT ( 'NONE',  ( 13.57481594606304576, 31.97109375216787441, -1.662435489736055892E-15 ) ) ;
#14461=CARTESIAN_POINT ( 'NONE',  ( -5.622872871577873077, 38.76757812500000000, 13.57481594606304753 ) ) ;
#14462=CARTESIAN_POINT ( 'NONE',  ( -8.312177448680279460E-16, 32.16953125216787157, -13.57481594606304576 ) ) ;
#14475=ORIENTED_EDGE ( 'NONE', *, *, #8803, .T. ) ;
#14501=CARTESIAN_POINT ( 'NONE',  ( 5.444914386472302859, 40.20625000108394431, 13.14518615778179189 ) ) ;
#14502=CARTESIAN_POINT ( 'NONE',  ( 9.598844408820459861, 39.01562500216787299, 9.598844408820456309 ) ) ;
#14513=EDGE_CURVE ( 'NONE', #3914, #22274, #15671, .T. ) ;
#14523=SHAPE_DEFINITION_REPRESENTATION ( #18345, #19878 ) ;
#14540=( BOUNDED_CURVE ( )  B_SPLINE_CURVE ( 2, ( #1069, #26867, #11293, #24716, #4914, #5194, #13574, #9738, #2773 ),
 .UNSPECIFIED., .F., .F. ) 
 B_SPLINE_CURVE_WITH_KNOTS ( ( 3, 2, 2, 2, 3 ),
 ( 0.4791666666666667962, 0.4895833333333333703, 0.5000000000000000000, 0.5104166666666665186, 0.5208333333333332593 ),
 .UNSPECIFIED. ) 
 CURVE ( )  GEOMETRIC_REPRESENTATION_ITEM ( )  RATIONAL_B_SPLINE_CURVE ( ( 0.9999999999999992228, 0.9238795325112875156, 1.000000000000000000, 0.9238795325112867385, 1.000000000000000000, 0.9238795325112867385, 1.000000000000000000, 0.9238795325112875156, 0.9999999999999992228 ) ) 
 REPRESENTATION_ITEM ( '' )  );
#14548=CARTESIAN_POINT ( 'NONE',  ( -13.14518615778179544, 38.96601562608393721, 0.000000000000000000 ) ) ;
#14564=CARTESIAN_POINT ( 'NONE',  ( 0.000000000000000000, 30.99999999999999645, 0.000000000000000000 ) ) ;
#14565=ORIENTED_EDGE ( 'NONE', *, *, #16531, .T. ) ;
#14577=FACE_OUTER_BOUND ( 'NONE', #1406, .T. ) ;
#14598=CARTESIAN_POINT ( 'NONE',  ( -13.14518615778179189, 32.07031250108393294, 5.444914386472304635 ) ) ;
#14599=CARTESIAN_POINT ( 'NONE',  ( 13.57481594606304753, 32.02070312716787015, -5.622872871577873077 ) ) ;
#14603=VECTOR ( 'NONE', #19185, 1000.000000000000000 ) ;
#14632=ORIENTED_EDGE ( 'NONE', *, *, #13327, .T. ) ;
#14635=CARTESIAN_POINT ( 'NONE',  ( 13.14518615778179900, 39.61093750108393863, -5.444914386472297529 ) ) ;
#14643=CARTESIAN_POINT ( 'NONE',  ( -8.312177448680279460E-16, 33.65781249999999147, -13.57481594606304576 ) ) ;
#14652=CARTESIAN_POINT ( 'NONE',  ( 5.444914386472302859, 40.00781250108393294, 13.14518615778179189 ) ) ;
#14677=CYLINDRICAL_SURFACE ( 'NONE', #4403, 13.57481594606304576 ) ;
#14688=CARTESIAN_POINT ( 'NONE',  ( 13.14518615778179900, 34.05468750108394005, -5.444914386472297529 ) ) ;
#14693=DIRECTION ( 'NONE',  ( 1.000000000000000000, 0.000000000000000000, 0.000000000000000000 ) ) ;
#14694=ORIENTED_EDGE ( 'NONE', *, *, #27950, .F. ) ;
#14695=CARTESIAN_POINT ( 'NONE',  ( -9.295050272127046043, 31.92148437608393508, -9.295050272127046043 ) ) ;
#14702=EDGE_CURVE ( 'NONE', #10337, #16728, #18095, .T. ) ;
#14707=FACE_OUTER_BOUND ( 'NONE', #21311, .T. ) ;
#14720=CARTESIAN_POINT ( 'NONE',  ( -13.14518615778179544, 40.75195312608393294, 0.000000000000000000 ) ) ;
#14723=CARTESIAN_POINT ( 'NONE',  ( -9.598844408820458085, 40.10703124999999147, -9.598844408820458085 ) ) ;
#14726=CYLINDRICAL_SURFACE ( 'NONE', #21835, 13.57481594606304576 ) ;
#14732=CARTESIAN_POINT ( 'NONE',  ( -5.622872871577873077, 40.35507812499998437, 13.57481594606304753 ) ) ;
#14733=CARTESIAN_POINT ( 'NONE',  ( 2.414731522848535132E-15, 39.95820312608393010, 13.14518615778179544 ) ) ;
#14743=CARTESIAN_POINT ( 'NONE',  ( -13.57481594606304398, 38.76757812716787299, 5.622872871577880183 ) ) ;
#14753=EDGE_LOOP ( 'NONE', ( #1355, #26805, #5775 ) ) ;
#14765=CARTESIAN_POINT ( 'NONE',  ( -9.598844408820458085, 40.90078124999999432, -9.598844408820458085 ) ) ;
#14770=CARTESIAN_POINT ( 'NONE',  ( 2.414731522848535132E-15, 38.56914062608393579, 13.14518615778179544 ) ) ;
#14771=CARTESIAN_POINT ( 'NONE',  ( 2.493653234604083739E-15, 39.71015625216787015, 13.57481594606304576 ) ) ;
#14778=ORIENTED_EDGE ( 'NONE', *, *, #21514, .T. ) ;
#14786=CARTESIAN_POINT ( 'NONE',  ( 13.14518615778179544, 38.56914062608393579, -1.609821015232357215E-15 ) ) ;
#14798=ORIENTED_EDGE ( 'NONE', *, *, #22894, .T. ) ;
#14812=CARTESIAN_POINT ( 'NONE',  ( 13.14518615778179544, 40.15664062608393436, -1.609821015232357215E-15 ) ) ;
#14813=CARTESIAN_POINT ( 'NONE',  ( 0.000000000000000000, 40.99999999999999289, 0.000000000000000000 ) ) ;
#14831=ORIENTED_EDGE ( 'NONE', *, *, #11147, .F. ) ;
#14860=CARTESIAN_POINT ( 'NONE',  ( -5.444914386472299306, 32.76484375108393010, 13.14518615778179722 ) ) ;
#14873=CARTESIAN_POINT ( 'NONE',  ( 5.622872871577878406, 38.86679687499999858, 13.57481594606304576 ) ) ;
#14874=CARTESIAN_POINT ( 'NONE',  ( -5.622872871577873077, 31.42539062716787157, -13.57481594606304753 ) ) ;
#14891=CARTESIAN_POINT ( 'NONE',  ( 1.907364849565526780E-15, 30.99999999999999645, 15.57481594606304576 ) ) ;
#14921=CARTESIAN_POINT ( 'NONE',  ( -8.312177448680279460E-16, 33.75703125216787726, -13.57481594606304576 ) ) ;
#14930=CARTESIAN_POINT ( 'NONE',  ( 2.414731522848535132E-15, 39.95820312608393010, 13.14518615778179544 ) ) ;
#14958=CARTESIAN_POINT ( 'NONE',  ( 13.14518615778179722, 37.03125000108393294, -5.444914386472297529 ) ) ;
#14965=CARTESIAN_POINT ( 'NONE',  ( 0.000000000000000000, 40.99999999999999289, 0.000000000000000000 ) ) ;
#14972=CARTESIAN_POINT ( 'NONE',  ( 0.000000000000000000, 40.99999999999999289, 0.000000000000000000 ) ) ;
#14977=CARTESIAN_POINT ( 'NONE',  ( -5.444914386472299306, 32.16953125108393152, 13.14518615778179722 ) ) ;
#14998=CARTESIAN_POINT ( 'NONE',  ( 2.414731522848535132E-15, 39.36289062608393152, 13.14518615778179544 ) ) ;
#15003=CARTESIAN_POINT ( 'NONE',  ( -9.295050272127046043, 39.85898437608393152, -9.295050272127046043 ) ) ;
#15008=VERTEX_POINT ( 'NONE', #21895 ) ;
#15010=CARTESIAN_POINT ( 'NONE',  ( 13.57481594606304753, 37.47773437500001137, -5.622872871577873077 ) ) ;
#15011=CARTESIAN_POINT ( 'NONE',  ( 9.295050272127046043, 36.28710937608393294, -9.295050272127046043 ) ) ;
#15048=CARTESIAN_POINT ( 'NONE',  ( 13.14518615778179900, 37.13046875108393863, 5.444914386472293977 ) ) ;
#15049=CARTESIAN_POINT ( 'NONE',  ( 13.57481594606304576, 36.73359375216787015, -1.662435489736055892E-15 ) ) ;
#15061=( NAMED_UNIT ( * ) PLANE_ANGLE_UNIT ( ) SI_UNIT ( $, .RADIAN. ) );
#15078=VERTEX_POINT ( 'NONE', #797 ) ;
#15085=CARTESIAN_POINT ( 'NONE',  ( -13.57481594606304576, 33.16171875216787868, 0.000000000000000000 ) ) ;
#15088=VERTEX_POINT ( 'NONE', #13590 ) ;
#15092=CARTESIAN_POINT ( 'NONE',  ( -8.049105076161786076E-16, 35.59257812608393579, -13.14518615778179544 ) ) ;
#15103=CARTESIAN_POINT ( 'NONE',  ( 0.000000000000000000, 40.99999999999999289, -13.57481594606304576 ) ) ;
#15109=CIRCLE ( 'NONE', #11951, 15.57481594606304576 ) ;
#15129=DIRECTION ( 'NONE',  ( 0.000000000000000000, 0.000000000000000000, -1.000000000000000000 ) ) ;
#15135=CARTESIAN_POINT ( 'NONE',  ( -8.049105076161786076E-16, 38.17226562608394147, -13.14518615778179544 ) ) ;
#15142=CARTESIAN_POINT ( 'NONE',  ( 5.444914386472297529, 37.32890625108393579, -13.14518615778179722 ) ) ;
#15149=CARTESIAN_POINT ( 'NONE',  ( 2.493653234604083739E-15, 37.22968749999999716, 13.57481594606304576 ) ) ;
#15150=CARTESIAN_POINT ( 'NONE',  ( 2.414731522848535132E-15, 38.37070312608393152, 13.14518615778179544 ) ) ;
#15185=DIRECTION ( 'NONE',  ( 0.000000000000000000, 1.000000000000000000, 0.000000000000000000 ) ) ;
#15186=CARTESIAN_POINT ( 'NONE',  ( 5.444914386472302859, 35.44375000108393436, 13.14518615778179189 ) ) ;
#15187=CARTESIAN_POINT ( 'NONE',  ( -5.622872871577873077, 36.98164062716787015, -13.57481594606304753 ) ) ;
#15196=VECTOR ( 'NONE', #5592, 1000.000000000000227 ) ;
#15199=CARTESIAN_POINT ( 'NONE',  ( 13.57481594606304931, 34.30273437716787299, 5.622872871577868636 ) ) ;
#15206=CARTESIAN_POINT ( 'NONE',  ( -5.444914386472299306, 39.90859375108393436, 13.14518615778179722 ) ) ;
#15213=CARTESIAN_POINT ( 'NONE',  ( -9.598844408820454532, 35.64218750216787868, 9.598844408820459861 ) ) ;
#15235=CARTESIAN_POINT ( 'NONE',  ( -9.295050272127044266, 35.09648437608392868, 9.295050272127047819 ) ) ;
#15237=EDGE_CURVE ( 'NONE', #27263, #58, #13490, .T. ) ;
#15280=ORIENTED_EDGE ( 'NONE', *, *, #16469, .F. ) ;
#15281=CARTESIAN_POINT ( 'NONE',  ( 5.444914386472302859, 37.82500000108392868, 13.14518615778179189 ) ) ;
#15287=CARTESIAN_POINT ( 'NONE',  ( -13.14518615778179544, 38.37070312608393152, 0.000000000000000000 ) ) ;
#15293=ORIENTED_EDGE ( 'NONE', *, *, #26043, .F. ) ;
#15294=CARTESIAN_POINT ( 'NONE',  ( -13.57481594606304753, 36.18789062499999432, -5.622872871577873077 ) ) ;
#15295=CARTESIAN_POINT ( 'NONE',  ( 2.414731522848535132E-15, 37.57695312608392868, 13.14518615778179544 ) ) ;
#15332=CARTESIAN_POINT ( 'NONE',  ( 5.444914386472302859, 37.03125000108393294, 13.14518615778179189 ) ) ;
#15333=CARTESIAN_POINT ( 'NONE',  ( -13.57481594606304576, 36.38632812716788578, 5.622872871577880183 ) ) ;
#15342=DIRECTION ( 'NONE',  ( -0.000000000000000000, -1.000000000000000000, -0.000000000000000000 ) ) ;
#15343=CARTESIAN_POINT ( 'NONE',  ( 5.622872871577961895, 34.50117187716787726, -13.57481594606295339 ) ) ;
#15351=CARTESIAN_POINT ( 'NONE',  ( 13.14518615778179900, 37.72578125108393721, 5.444914386472293977 ) ) ;
#15380=CARTESIAN_POINT ( 'NONE',  ( -9.295050272127046043, 35.69179687608393436, -9.295050272127046043 ) ) ;
#15424=CARTESIAN_POINT ( 'NONE',  ( 5.444914386472302859, 39.41250000108393436, 13.14518615778179189 ) ) ;
#15430=CARTESIAN_POINT ( 'NONE',  ( -13.14518615778179189, 37.62656250108393152, 5.444914386472304635 ) ) ;
#15431=CARTESIAN_POINT ( 'NONE',  ( -5.622872871577947684, 39.36289062716787157, -13.57481594606297293 ) ) ;
#15437=CARTESIAN_POINT ( 'NONE',  ( 13.57481594606304576, 35.84062499999999574, -1.662435489736055892E-15 ) ) ;
#15438=CARTESIAN_POINT ( 'NONE',  ( 13.14518615778179900, 36.13828125108393863, 5.444914386472293977 ) ) ;
#15454=DIRECTION ( 'NONE',  ( 0.000000000000000000, 0.000000000000000000, 1.000000000000000000 ) ) ;
#15468=CARTESIAN_POINT ( 'NONE',  ( -9.598844408820454532, 39.51171874999999289, 9.598844408820459861 ) ) ;
#15469=CARTESIAN_POINT ( 'NONE',  ( 2.493653234604083739E-15, 39.71015625216787015, 13.57481594606304576 ) ) ;
#15474=CARTESIAN_POINT ( 'NONE',  ( 13.14518615778179900, 37.92421875108392726, 5.444914386472293977 ) ) ;
#15475=CARTESIAN_POINT ( 'NONE',  ( 13.57481594606304576, 35.93984375216787441, -1.662435489736055892E-15 ) ) ;
#15483=CARTESIAN_POINT ( 'NONE',  ( 1.662435489736055892E-15, 40.99999999999999289, 13.57481594606304576 ) ) ;
#15486=DIRECTION ( 'NONE',  ( 0.000000000000000000, 0.000000000000000000, -1.000000000000000000 ) ) ;
#15491=( BOUNDED_CURVE ( )  B_SPLINE_CURVE ( 2, ( #28166, #89, #8770, #2508, #12880, #17602, #8911, #19467, #17459 ),
 .UNSPECIFIED., .F., .F. ) 
 B_SPLINE_CURVE_WITH_KNOTS ( ( 3, 2, 2, 2, 3 ),
 ( 0.3958333333333331483, 0.4062499999999999445, 0.4166666666666667407, 0.4270833333333335369, 0.4375000000000003331 ),
 .UNSPECIFIED. ) 
 CURVE ( )  GEOMETRIC_REPRESENTATION_ITEM ( )  RATIONAL_B_SPLINE_CURVE ( ( 1.000000000000001110, 0.9238795325112855172, 1.000000000000000000, 0.9238795325112867385, 1.000000000000000000, 0.9238795325112867385, 1.000000000000000000, 0.9238795325112842960, 1.000000000000002442 ) ) 
 REPRESENTATION_ITEM ( '' )  );
#15493=B_SPLINE_CURVE_WITH_KNOTS ( 'NONE', 3,
 ( #25504, #22963, #27516, #3425 ),
 .UNSPECIFIED., .F., .F.,
 ( 4, 4 ),
 ( 0.000000000000000000, 1.000000000000000000 ),
 .UNSPECIFIED. ) ;
#15498=CARTESIAN_POINT ( 'NONE',  ( -5.444914386472297529, 35.64218750108392442, -13.14518615778179900 ) ) ;
#15500=VECTOR ( 'NONE', #13772, 1000.000000000000000 ) ;
#15502=DIRECTION ( 'NONE',  ( 0.000000000000000000, 1.000000000000000000, 0.000000000000000000 ) ) ;
#15526=UNCERTAINTY_MEASURE_WITH_UNIT (LENGTH_MEASURE( 1.000000000000000082E-05 ), #1949, 'distance_accuracy_value', 'NONE');
#15528=CARTESIAN_POINT ( 'NONE',  ( 9.295050272127046043, 36.28710937608393294, -9.295050272127046043 ) ) ;
#15565=VECTOR ( 'NONE', #25500, 1000.000000000000000 ) ;
#15570=CARTESIAN_POINT ( 'NONE',  ( -13.14518615778179189, 38.42031250108393436, 5.444914386472304635 ) ) ;
#15576=CARTESIAN_POINT ( 'NONE',  ( 9.295050272127047819, 37.87460937608393863, 9.295050272127046043 ) ) ;
#15582=CARTESIAN_POINT ( 'NONE',  ( -8.312177448680279460E-16, 35.24531249999999716, -13.57481594606304576 ) ) ;
#15583=CARTESIAN_POINT ( 'NONE',  ( 9.295050272127046043, 37.08085937608393579, -9.295050272127046043 ) ) ;
#15601=SURFACE_STYLE_FILL_AREA ( #22607 ) ;
#15617=DIRECTION ( 'NONE',  ( 0.000000000000000000, 1.000000000000000000, 0.000000000000000000 ) ) ;
#15624=CARTESIAN_POINT ( 'NONE',  ( -13.14518615778179189, 36.83281250108393579, 5.444914386472304635 ) ) ;
#15625=CARTESIAN_POINT ( 'NONE',  ( 5.622872871577871301, 38.46992187716787015, -13.57481594606304753 ) ) ;
#15640=( LENGTH_UNIT ( ) NAMED_UNIT ( * ) SI_UNIT ( .MILLI., .METRE. ) );
#15647=CARTESIAN_POINT ( 'NONE',  ( -8.049105076161786076E-16, 37.18007812608393436, -13.14518615778179544 ) ) ;
#15663=CARTESIAN_POINT ( 'NONE',  ( 5.622872871577786924, 34.10429687500000284, 13.57481594606313813 ) ) ;
#15671=( BOUNDED_CURVE ( )  B_SPLINE_CURVE ( 2, ( #23391, #21112, #26081, #1876, #15085, #21674, #3864, #12673, #6141 ),
 .UNSPECIFIED., .F., .T. ) 
 B_SPLINE_CURVE_WITH_KNOTS ( ( 3, 2, 2, 2, 3 ),
 ( 0.7291666666666668517, 0.7395833333333334814, 0.7500000000000001110, 0.7604166666666667407, 0.7708333333333333703 ),
 .UNSPECIFIED. ) 
 CURVE ( )  GEOMETRIC_REPRESENTATION_ITEM ( )  RATIONAL_B_SPLINE_CURVE ( ( 0.9999999999999983347, 0.9238795325112884038, 1.000000000000000000, 0.9238795325112867385, 1.000000000000000000, 0.9238795325112867385, 1.000000000000000000, 0.9238795325112867385, 1.000000000000000000 ) ) 
 REPRESENTATION_ITEM ( '' )  );
#15674=CARTESIAN_POINT ( 'NONE',  ( 13.14518615778179722, 32.16953125108393152, 5.444914386472293977 ) ) ;
#15691=EDGE_LOOP ( 'NONE', ( #5138, #1734, #12355, #263 ) ) ;
#15714=CARTESIAN_POINT ( 'NONE',  ( 2.414731522848535132E-15, 34.60039062608393579, 13.14518615778179544 ) ) ;
#15720=CARTESIAN_POINT ( 'NONE',  ( -9.295050272127046043, 39.06523437608392868, -9.295050272127046043 ) ) ;
#15726=CARTESIAN_POINT ( 'NONE',  ( 13.57481594606304576, 32.66562499999999858, -1.662435489736055892E-15 ) ) ;
#15727=CARTESIAN_POINT ( 'NONE',  ( 2.414731522848535132E-15, 35.19570312608392726, 13.14518615778179544 ) ) ;
#15737=EDGE_CURVE ( 'NONE', #8402, #26359, #25181, .T. ) ;
#15741=CARTESIAN_POINT ( 'NONE',  ( -5.622872871577782483, 34.60039062716787583, -13.57481594606313990 ) ) ;
#15763=CARTESIAN_POINT ( 'NONE',  ( -9.295050272127046043, 32.71523437608393436, -9.295050272127046043 ) ) ;
#15764=CARTESIAN_POINT ( 'NONE',  ( 13.57481594606304931, 35.09648437716787583, 5.622872871577869525 ) ) ;
#15788=CARTESIAN_POINT ( 'NONE',  ( 5.444914386472297529, 34.74921875108394431, -13.14518615778179900 ) ) ;
#15807=ADVANCED_BREP_SHAPE_REPRESENTATION ( '', ( #17477, #26844 ), #9975 ) ;
#15815=CARTESIAN_POINT ( 'NONE',  ( 2.414731522848535132E-15, 34.40195312608393152, 13.14518615778179544 ) ) ;
#15831=EDGE_LOOP ( 'NONE', ( #9395, #21851 ) ) ;
#15855=CARTESIAN_POINT ( 'NONE',  ( 5.444914386472302859, 37.03125000108393294, 13.14518615778179189 ) ) ;
#15860=CARTESIAN_POINT ( 'NONE',  ( -5.444914386472299306, 34.55078125108393294, 13.14518615778179722 ) ) ;
#15866=CARTESIAN_POINT ( 'NONE',  ( 13.57481594606304576, 34.25312499999999716, -1.662435489736055892E-15 ) ) ;
#15867=CARTESIAN_POINT ( 'NONE',  ( 2.414731522848535132E-15, 34.40195312608393152, 13.14518615778179544 ) ) ;
#15868=ORIENTED_EDGE ( 'NONE', *, *, #27428, .T. ) ;
#15872=ORIENTED_EDGE ( 'NONE', *, *, #13151, .T. ) ;
#15898=CARTESIAN_POINT ( 'NONE',  ( -9.295050272127046043, 34.30273437608393294, -9.295050272127046043 ) ) ;
#15899=CARTESIAN_POINT ( 'NONE',  ( -13.57481594606304576, 33.21132812716787441, 5.622872871577880183 ) ) ;
#15912=CARTESIAN_POINT ( 'NONE',  ( -13.57481594606304576, 40.30546875216787583, 0.000000000000000000 ) ) ;
#15921=CARTESIAN_POINT ( 'NONE',  ( -8.049105076161786076E-16, 36.38632812608393152, -13.14518615778179544 ) ) ;
#15952=CARTESIAN_POINT ( 'NONE',  ( 5.444914386472302859, 33.65781250108393152, 13.14518615778179189 ) ) ;
#15968=FACE_OUTER_BOUND ( 'NONE', #6270, .T. ) ;
#15970=EDGE_LOOP ( 'NONE', ( #20840, #14424, #10622, #17430 ) ) ;
#15991=ORIENTED_EDGE ( 'NONE', *, *, #18231, .F. ) ;
#15992=CARTESIAN_POINT ( 'NONE',  ( 13.14518615778179544, 34.79882812608394005, -1.609821015232357215E-15 ) ) ;
#15998=CARTESIAN_POINT ( 'NONE',  ( 13.14518615778179722, 33.95546875108394147, 5.444914386472293977 ) ) ;
#16006=CARTESIAN_POINT ( 'NONE',  ( 2.493653234604083739E-15, 32.46718749999999432, 13.57481594606304576 ) ) ;
#16007=CARTESIAN_POINT ( 'NONE',  ( 5.444914386472302859, 32.86406250108392868, 13.14518615778179189 ) ) ;
#16022=ORIENTED_EDGE ( 'NONE', *, *, #26189, .F. ) ;
#16034=( BOUNDED_CURVE ( )  B_SPLINE_CURVE ( 2, ( #4183, #8729, #19424, #21857, #2469, #4464, #8870, #23845, #17849 ),
 .UNSPECIFIED., .F., .F. ) 
 B_SPLINE_CURVE_WITH_KNOTS ( ( 3, 2, 2, 2, 3 ),
 ( 0.6874999999999997780, 0.6979166666666665186, 0.7083333333333333703, 0.7187500000000001110, 0.7291666666666668517 ),
 .UNSPECIFIED. ) 
 CURVE ( )  GEOMETRIC_REPRESENTATION_ITEM ( )  RATIONAL_B_SPLINE_CURVE ( ( 1.000000000000001554, 0.9238795325112850731, 1.000000000000000000, 0.9238795325112867385, 1.000000000000000000, 0.9238795325112867385, 1.000000000000000000, 0.9238795325112850731, 1.000000000000001554 ) ) 
 REPRESENTATION_ITEM ( '' )  );
#16042=CARTESIAN_POINT ( 'NONE',  ( 13.14518615778179544, 34.79882812608394005, -1.609821015232357215E-15 ) ) ;
#16043=CARTESIAN_POINT ( 'NONE',  ( 5.622872871577878406, 34.99726562716787726, 13.57481594606304576 ) ) ;
#16057=CYLINDRICAL_SURFACE ( 'NONE', #1541, 13.57481594606304576 ) ;
#16065=CARTESIAN_POINT ( 'NONE',  ( -8.312177448680279460E-16, 40.80156249999999574, -13.57481594606304576 ) ) ;
#16067=CARTESIAN_POINT ( 'NONE',  ( -9.295050272127046043, 33.31054687608393294, -9.295050272127046043 ) ) ;
#16070=CARTESIAN_POINT ( 'NONE',  ( -13.57481594606304753, 37.87460937716787868, -5.622872871577872189 ) ) ;
#16074=CARTESIAN_POINT ( 'NONE',  ( -13.57481594606304576, 35.54296875216788010, 0.000000000000000000 ) ) ;
#16096=CARTESIAN_POINT ( 'NONE',  ( 5.444914386472302859, 34.45156250108392726, 13.14518615778179189 ) ) ;
#16113=DIRECTION ( 'NONE',  ( 0.000000000000000000, 0.000000000000000000, -1.000000000000000000 ) ) ;
#16124=EDGE_CURVE ( 'NONE', #17847, #58, #11634, .T. ) ;
#16141=CARTESIAN_POINT ( 'NONE',  ( 9.295050272127047819, 35.49335937608393721, 9.295050272127046043 ) ) ;
#16146=CARTESIAN_POINT ( 'NONE',  ( -13.14518615778179722, 35.14609375108393152, -5.444914386472297529 ) ) ;
#16153=CARTESIAN_POINT ( 'NONE',  ( -13.57481594606304576, 33.85624999999999574, 0.000000000000000000 ) ) ;
#16154=CARTESIAN_POINT ( 'NONE',  ( -5.444914386472299306, 34.35234375108392868, 13.14518615778179722 ) ) ;
#16184=CARTESIAN_POINT ( 'NONE',  ( -8.312177448680279460E-16, 35.34453125216787583, -13.57481594606304576 ) ) ;
#16190=CARTESIAN_POINT ( 'NONE',  ( 9.295050272127047819, 34.69960937608393436, 9.295050272127046043 ) ) ;
#16191=CARTESIAN_POINT ( 'NONE',  ( 13.57481594606304931, 32.71523437716787441, 5.622872871577869525 ) ) ;
#16215=CARTESIAN_POINT ( 'NONE',  ( 9.295050272127046043, 33.11210937608393579, -9.295050272127046043 ) ) ;
#16223=VECTOR ( 'NONE', #11646, 1000.000000000000000 ) ;
#16246=CARTESIAN_POINT ( 'NONE',  ( -13.14518615778179189, 31.87187500108393223, 5.444914386472304635 ) ) ;
#16285=CARTESIAN_POINT ( 'NONE',  ( -5.444914386472297529, 31.87187500108393223, -13.14518615778179900 ) ) ;
#16292=CARTESIAN_POINT ( 'NONE',  ( -9.295050272127046043, 35.89023437608393152, -9.295050272127046043 ) ) ;
#16299=CARTESIAN_POINT ( 'NONE',  ( -13.57481594606304753, 32.21914062500000142, -5.622872871577873077 ) ) ;
#16300=CARTESIAN_POINT ( 'NONE',  ( 9.295050272127046043, 33.90585937608393152, -9.295050272127046043 ) ) ;
#16306=CARTESIAN_POINT ( 'NONE',  ( 0.000000000000000000, 40.99999999999999289, -13.57481594606304576 ) ) ;
#16336=CARTESIAN_POINT ( 'NONE',  ( -9.295050272127044266, 34.50117187608393721, 9.295050272127047819 ) ) ;
#16337=CARTESIAN_POINT ( 'NONE',  ( 2.493653234604083739E-15, 34.15390625216787157, 13.57481594606304576 ) ) ;
#16359=CARTESIAN_POINT ( 'NONE',  ( 13.14518615778179900, 32.96328125108393436, 5.444914386472293977 ) ) ;
#16362=CARTESIAN_POINT ( 'NONE',  ( -13.57481594606304398, 37.97382812716787726, 5.622872871577880183 ) ) ;
#16370=EDGE_LOOP ( 'NONE', ( #8702, #9117, #8363, #10944, #20420, #16883, #16514, #13224, #14114, #16022, #13401, #13572, #4673, #5964, #6446, #27416, #4555, #1609, #18100, #3519, #13787, #11983, #2077, #2607, #15991, #25082, #22277 ) ) ;
#16400=VECTOR ( 'NONE', #6705, 1000.000000000000000 ) ;
#16407=EDGE_LOOP ( 'NONE', ( #8052, #13188, #16787, #10482 ) ) ;
#16418=CARTESIAN_POINT ( 'NONE',  ( 13.14518615778179544, 38.56914062608393579, -1.609821015232357215E-15 ) ) ;
#16425=CARTESIAN_POINT ( 'NONE',  ( 13.14518615778179900, 33.16171875108393863, 5.444914386472293977 ) ) ;
#16429=CARTESIAN_POINT ( 'NONE',  ( 9.598844408820456309, 39.21406250216787015, -9.598844408820458085 ) ) ;
#16431=CARTESIAN_POINT ( 'NONE',  ( 5.444914386472297529, 35.74140625108393721, -13.14518615778179722 ) ) ;
#16441=CARTESIAN_POINT ( 'NONE',  ( 13.57481594606304753, 32.81445312716787299, -5.622872871577873966 ) ) ;
#16443=EDGE_CURVE ( 'NONE', #6267, #2719, #4086, .T. ) ;
#16447=CARTESIAN_POINT ( 'NONE',  ( -13.57481594606304753, 33.80664062499999289, -5.622872871577872189 ) ) ;
#16453=ORIENTED_EDGE ( 'NONE', *, *, #2373, .F. ) ;
#16458=CARTESIAN_POINT ( 'NONE',  ( -5.622872871577890841, 40.35507812499999147, 13.57481594606302444 ) ) ;
#16469=EDGE_CURVE ( 'NONE', #9928, #24154, #14294, .T. ) ;
#16472=CARTESIAN_POINT ( 'NONE',  ( -13.57481594606304576, 38.61874999999999147, 0.000000000000000000 ) ) ;
#16473=CARTESIAN_POINT ( 'NONE',  ( 9.295050272127046043, 40.25585937608393294, -9.295050272127046043 ) ) ;
#16477=ORIENTED_EDGE ( 'NONE', *, *, #22954, .T. ) ;
#16493=DIRECTION ( 'NONE',  ( -0.000000000000000000, -1.000000000000000000, -0.000000000000000000 ) ) ;
#16499=CARTESIAN_POINT ( 'NONE',  ( 6.944426393311538881, 31.55306875057403104, -11.16113171639042356 ) ) ;
#16514=ORIENTED_EDGE ( 'NONE', *, *, #6390, .F. ) ;
#16525=ORIENTED_EDGE ( 'NONE', *, *, #12453, .F. ) ;
#16531=EDGE_CURVE ( 'NONE', #22274, #17326, #6760, .T. ) ;
#16545=CARTESIAN_POINT ( 'NONE',  ( 5.622872871577796694, 39.95820312499999716, -13.57481594606312036 ) ) ;
#16553=( BOUNDED_CURVE ( )  B_SPLINE_CURVE ( 2, ( #16836, #14268, #25533, #12121, #16560, #22987, #10407, #25398, #14812, #3456, #3737, #3870, #10261, #16699, #19114, #18971, #27679, #27821, #8142, #1326, #5878, #8275, #3600, #16965, #25665, #18702, #10122, #1883, #27270, #12397, #27405, #21260, #14548, #23537, #7866, #1742, #20985, #18835, #23397, #5741, #16418, #4013, #21118, #25251, #12679, #23263, #7999, #23125, #14409, #21405, #10546, #1466, #7726, #25115, #1605, #21827, #300, #17675, #17248, #21682, #4154, #26382, #28094, #17390, #10818, #13087, #8557, #22106, #27955, #2302, #2442, #14958, #21965, #19673, #11103, #15, #10962, #12814, #21537, #17101, #4718, #8412, #158, #25949, #19533, #19817, #15528, #23677, #2014, #19254, #12948, #10682, #26089, #24235, #19389, #25804, #6423, #13377, #15380, #23812, #15092, #2585, #8841, #4289, #6837, #2158, #8985, #6281, #8699, #6555, #15235, #23955, #17532, #4435, #26234, #6692, #24095, #4571, #13231, #7402, #2725, #24374, #24943, #16096, #15815, #13528, #13950, #24803, #11671, #9264, #14098, #2998, #22817, #5285, #20538, #11244, #17818, #24521, #24666, #15952, #27098, #2858, #4863, #5142, #26959, #20392, #22248, #878, #11388, #6978, #5007, #19963, #441, #20109, #20244, #26523, #11526, #13808, #9549, #11816, #26814, #22676, #22530, #729, #3149, #18251, #1021, #9692, #18392, #15674, #9402, #9125, #22386, #586, #7550, #16246, #5429, #18101, #17960, #13670, #26670, #7117, #7261 ),
 .UNSPECIFIED., .F., .F. ) 
 B_SPLINE_CURVE_WITH_KNOTS ( ( 3, 2, 2, 2, 2, 2, 2, 2, 2, 2, 2, 2, 2, 2, 2, 2, 2, 2, 2, 2, 2, 2, 2, 2, 2, 2, 2, 2, 2, 2, 2, 2, 2, 2, 2, 2, 2, 2, 2, 2, 2, 2, 2, 2, 2, 2, 2, 2, 2, 2, 2, 2, 2, 2, 2, 2, 2, 2, 2, 2, 2, 2, 2, 2, 2, 2, 2, 2, 2, 2, 2, 2, 2, 2, 2, 2, 2, 2, 2, 2, 2, 2, 2, 2, 2, 2, 2, 2, 2, 2, 2, 3 ),
 ( 0.000000000000000000, 0.01041666666666666609, 0.02083333333333333218, 0.03125000000000000000, 0.04166666666666666435, 0.05208333333333332871, 0.06250000000000000000, 0.07291666666666667129, 0.08333333333333332871, 0.09375000000000000000, 0.1041666666666666574, 0.1145833333333333287, 0.1250000000000000000, 0.1354166666666666574, 0.1458333333333333426, 0.1562500000000000000, 0.1666666666666666574, 0.1770833333333333426, 0.1875000000000000000, 0.1979166666666666574, 0.2083333333333333148, 0.2187500000000000000, 0.2291666666666666574, 0.2395833333333333426, 0.2500000000000000000, 0.2604166666666666852, 0.2708333333333333148, 0.2812500000000000000, 0.2916666666666666852, 0.3020833333333333148, 0.3125000000000000000, 0.3229166666666666852, 0.3333333333333333148, 0.3437500000000000000, 0.3541666666666666852, 0.3645833333333333148, 0.3750000000000000000, 0.3854166666666666852, 0.3958333333333333148, 0.4062500000000000000, 0.4166666666666666297, 0.4270833333333333148, 0.4375000000000000000, 0.4479166666666666852, 0.4583333333333333148, 0.4687500000000000000, 0.4791666666666666852, 0.4895833333333333148, 0.5000000000000000000, 0.5104166666666666297, 0.5208333333333333703, 0.5312500000000000000, 0.5416666666666666297, 0.5520833333333333703, 0.5625000000000000000, 0.5729166666666665186, 0.5833333333333333703, 0.5937500000000000000, 0.6041666666666666297, 0.6145833333333333703, 0.6250000000000000000, 0.6354166666666666297, 0.6458333333333333703, 0.6562500000000000000, 0.6666666666666666297, 0.6770833333333333703, 0.6875000000000000000, 0.6979166666666666297, 0.7083333333333333703, 0.7187500000000000000, 0.7291666666666666297, 0.7395833333333333703, 0.7500000000000000000, 0.7604166666666666297, 0.7708333333333333703, 0.7812500000000000000, 0.7916666666666666297, 0.8020833333333333703, 0.8125000000000000000, 0.8229166666666666297, 0.8333333333333332593, 0.8437500000000000000, 0.8541666666666666297, 0.8645833333333333703, 0.8750000000000000000, 0.8854166666666666297, 0.8958333333333333703, 0.9062500000000000000, 0.9166666666666666297, 0.9270833333333333703, 0.9375000000000000000, 0.9448586970929392370 ),
 .UNSPECIFIED. ) 
 CURVE ( )  GEOMETRIC_REPRESENTATION_ITEM ( )  RATIONAL_B_SPLINE_CURVE ( ( 1.000000000000000000, 0.9238795325112867385, 1.000000000000000000, 0.9238795325112867385, 1.000000000000000000, 0.9238795325112867385, 1.000000000000000000, 0.9238795325112867385, 1.000000000000000000, 0.9238795325112867385, 1.000000000000000000, 0.9238795325112867385, 1.000000000000000000, 0.9238795325112867385, 1.000000000000000000, 0.9238795325112867385, 1.000000000000000000, 0.9238795325112867385, 1.000000000000000000, 0.9238795325112867385, 1.000000000000000000, 0.9238795325112867385, 1.000000000000000000, 0.9238795325112867385, 1.000000000000000000, 0.9238795325112867385, 1.000000000000000000, 0.9238795325112867385, 1.000000000000000000, 0.9238795325112867385, 1.000000000000000000, 0.9238795325112867385, 1.000000000000000000, 0.9238795325112867385, 1.000000000000000000, 0.9238795325112867385, 1.000000000000000000, 0.9238795325112867385, 1.000000000000000000, 0.9238795325112867385, 1.000000000000000000, 0.9238795325112867385, 1.000000000000000000, 0.9238795325112867385, 1.000000000000000000, 0.9238795325112867385, 1.000000000000000000, 0.9238795325112867385, 1.000000000000000000, 0.9238795325112867385, 1.000000000000000000, 0.9238795325112867385, 1.000000000000000000, 0.9238795325112867385, 1.000000000000000000, 0.9238795325112867385, 1.000000000000000000, 0.9238795325112867385, 1.000000000000000000, 0.9238795325112867385, 1.000000000000000000, 0.9238795325112867385, 1.000000000000000000, 0.9238795325112867385, 1.000000000000000000, 0.9238795325112867385, 1.000000000000000000, 0.9238795325112867385, 1.000000000000000000, 0.9238795325112867385, 1.000000000000000000, 0.9238795325112867385, 1.000000000000000000, 0.9238795325112867385, 1.000000000000000000, 0.9238795325112867385, 1.000000000000000000, 0.9238795325112867385, 1.000000000000000000, 0.9238795325112867385, 1.000000000000000000, 0.9238795325112867385, 1.000000000000000000, 0.9238795325112867385, 1.000000000000000000, 0.9238795325112867385, 1.000000000000000000, 0.9238795325112867385, 1.000000000000000000, 0.9238795325112867385, 1.000000000000000000, 0.9238795325112867385, 1.000000000000000000, 0.9238795325112867385, 1.000000000000000000, 0.9238795325112867385, 1.000000000000000000, 0.9238795325112867385, 1.000000000000000000, 0.9238795325112867385, 1.000000000000000000, 0.9238795325112867385, 1.000000000000000000, 0.9238795325112867385, 1.000000000000000000, 0.9238795325112867385, 1.000000000000000000, 0.9238795325112867385, 1.000000000000000000, 0.9238795325112867385, 1.000000000000000000, 0.9238795325112867385, 1.000000000000000000, 0.9238795325112867385, 1.000000000000000000, 0.9238795325112867385, 1.000000000000000000, 0.9238795325112867385, 1.000000000000000000, 0.9238795325112867385, 1.000000000000000000, 0.9238795325112867385, 1.000000000000000000, 0.9238795325112867385, 1.000000000000000000, 0.9238795325112867385, 1.000000000000000000, 0.9238795325112867385, 1.000000000000000000, 0.9238795325112867385, 1.000000000000000000, 0.9238795325112867385, 1.000000000000000000, 0.9238795325112867385, 1.000000000000000000, 0.9238795325112867385, 1.000000000000000000, 0.9238795325112867385, 1.000000000000000000, 0.9238795325112867385, 1.000000000000000000, 0.9238795325112867385, 1.000000000000000000, 0.9238795325112867385, 1.000000000000000000, 0.9238795325112867385, 1.000000000000000000, 0.9238795325112867385, 1.000000000000000000, 0.9238795325112867385, 1.000000000000000000, 0.9238795325112867385, 1.000000000000000000, 0.9238795325112867385, 1.000000000000000000, 0.9238795325112867385, 1.000000000000000000, 0.9238795325112867385, 1.000000000000000000, 0.9238795325112867385, 1.000000000000000000, 0.9238795325112867385, 1.000000000000000000, 0.9238795325112867385, 1.000000000000000000, 0.9238795325112867385, 1.000000000000000000, 0.9238795325112867385, 1.000000000000000000, 0.9238795325112867385, 1.000000000000000000, 0.9238795325112867385, 1.000000000000000000, 0.9238795325112867385, 1.000000000000000000, 0.9238795325112867385, 1.000000000000000000, 0.9238795325112867385, 1.000000000000000000, 0.9238795325112867385, 1.000000000000000000, 0.9462258435690522607, 0.9684275710300105366 ) ) 
 REPRESENTATION_ITEM ( '' )  );
#16560=CARTESIAN_POINT ( 'NONE',  ( -8.049105076161786076E-16, 40.35507812608393152, -13.14518615778179544 ) ) ;
#16567=CARTESIAN_POINT ( 'NONE',  ( -13.14518615778179189, 32.86406250108393579, 5.444914386472304635 ) ) ;
#16573=CARTESIAN_POINT ( 'NONE',  ( -13.14518615778179722, 32.76484375108393010, -5.444914386472297529 ) ) ;
#16581=CARTESIAN_POINT ( 'NONE',  ( -13.14518615778179544, 31.82226562608393650, 0.000000000000000000 ) ) ;
#16585=CARTESIAN_POINT ( 'NONE',  ( 13.57481594606304576, 35.04687499999999289, -1.662435489736055892E-15 ) ) ;
#16594=CARTESIAN_POINT ( 'NONE',  ( 13.57481594606304753, 32.02070312716787015, -5.622872871577873966 ) ) ;
#16597=VERTEX_POINT ( 'NONE', #20871 ) ;
#16612=CARTESIAN_POINT ( 'NONE',  ( -5.622872871577965448, 37.27929687716785878, 13.57481594606295161 ) ) ;
#16614=CARTESIAN_POINT ( 'NONE',  ( 6.944423624769117787, 31.75150628229955529, -11.16113343896966370 ) ) ;
#16615=CARTESIAN_POINT ( 'NONE',  ( -13.14518615778179544, 40.55351562608393579, 0.000000000000000000 ) ) ;
#16624=CARTESIAN_POINT ( 'NONE',  ( 0.000000000000000000, 40.99999999999999289, 0.000000000000000000 ) ) ;
#16633=LINE ( 'NONE', #1403, #4049 ) ;
#16654=CARTESIAN_POINT ( 'NONE',  ( 9.295050272127046043, 40.45429687608393721, -9.295050272127046043 ) ) ;
#16655=CARTESIAN_POINT ( 'NONE',  ( 13.57481594606304576, 39.11484375216787157, -1.662435489736055892E-15 ) ) ;
#16671=CARTESIAN_POINT ( 'NONE',  ( 2.493653234604083739E-15, 34.05468749999999289, 13.57481594606304576 ) ) ;
#16692=ADVANCED_FACE ( 'NONE', ( #14707 ), #23564, .T. ) ;
#16699=CARTESIAN_POINT ( 'NONE',  ( -5.444914386472299306, 39.90859375108392726, 13.14518615778179722 ) ) ;
#16709=CARTESIAN_POINT ( 'NONE',  ( 2.414731522848535132E-15, 32.21914062608393436, 13.14518615778179544 ) ) ;
#16723=CARTESIAN_POINT ( 'NONE',  ( 2.493653234604083739E-15, 32.46718749999999432, 13.57481594606304576 ) ) ;
#16727=CARTESIAN_POINT ( 'NONE',  ( 9.598844408820459861, 34.94765624999999432, 9.598844408820456309 ) ) ;
#16728=VERTEX_POINT ( 'NONE', #19285 ) ;
#16731=CARTESIAN_POINT ( 'NONE',  ( -5.622872871577965448, 34.00507812499998295, 13.57481594606295161 ) ) ;
#16743=CARTESIAN_POINT ( 'NONE',  ( 13.14518615778179722, 39.61093750108393863, -5.444914386472297529 ) ) ;
#16749=CARTESIAN_POINT ( 'NONE',  ( 5.622872871577878406, 40.45429687500001137, 13.57481594606304576 ) ) ;
#16750=CARTESIAN_POINT ( 'NONE',  ( 2.414731522848535132E-15, 39.16445312608392726, 13.14518615778179544 ) ) ;
#16768=CARTESIAN_POINT ( 'NONE',  ( 1.662435489736055892E-15, 40.99999999999999289, 13.57481594606304576 ) ) ;
#16771=CARTESIAN_POINT ( 'NONE',  ( -13.57481594606304753, 32.31835937716787299, -5.622872871577872189 ) ) ;
#16787=ORIENTED_EDGE ( 'NONE', *, *, #26334, .T. ) ;
#16789=CARTESIAN_POINT ( 'NONE',  ( 5.444914386472297529, 40.50390625108394005, -13.14518615778179900 ) ) ;
#16808=CARTESIAN_POINT ( 'NONE',  ( -5.444914386472297529, 38.81718750108393579, -13.14518615778179900 ) ) ;
#16836=CARTESIAN_POINT ( 'NONE',  ( -13.14518615778179544, 40.55351562608393579, 0.000000000000000000 ) ) ;
#16846=CARTESIAN_POINT ( 'NONE',  ( 13.14518615778179900, 33.26093750108393721, -5.444914386472297529 ) ) ;
#16851=DIRECTION ( 'NONE',  ( 0.000000000000000000, 1.000000000000000000, 0.000000000000000000 ) ) ;
#16853=CARTESIAN_POINT ( 'NONE',  ( 13.14518615778179722, 32.46718750108393436, -5.444914386472297529 ) ) ;
#16858=CARTESIAN_POINT ( 'NONE',  ( -13.57481594606304753, 32.21914062499999432, -5.622872871577872189 ) ) ;
#16883=ORIENTED_EDGE ( 'NONE', *, *, #9667, .F. ) ;
#16884=CARTESIAN_POINT ( 'NONE',  ( -8.312177448680279460E-16, 39.21406249999999716, -13.57481594606304576 ) ) ;
#16885=CARTESIAN_POINT ( 'NONE',  ( -13.57481594606304576, 32.41757812716787157, 5.622872871577880183 ) ) ;
#16921=CARTESIAN_POINT ( 'NONE',  ( 13.14518615778179900, 38.71796875108393721, 5.444914386472293977 ) ) ;
#16922=CARTESIAN_POINT ( 'NONE',  ( -13.57481594606304753, 40.25585937716787299, -5.622872871577873077 ) ) ;
#16937=CARTESIAN_POINT ( 'NONE',  ( 2.414731522848535132E-15, 38.37070312608393152, 13.14518615778179544 ) ) ;
#16948=ORIENTED_EDGE ( 'NONE', *, *, #1313, .F. ) ;
#16965=CARTESIAN_POINT ( 'NONE',  ( 13.14518615778179722, 39.41250000108393436, -5.444914386472297529 ) ) ;
#16971=ORIENTED_EDGE ( 'NONE', *, *, #26189, .T. ) ;
#17005=CARTESIAN_POINT ( 'NONE',  ( 5.444914386472297529, 33.16171875108393152, -13.14518615778179900 ) ) ;
#17017=CARTESIAN_POINT ( 'NONE',  ( 13.57481594606304753, 39.06523437499998863, -5.622872871577873077 ) ) ;
#17018=CARTESIAN_POINT ( 'NONE',  ( -9.598844408820454532, 31.67343750216787512, 9.598844408820459861 ) ) ;
#17055=CARTESIAN_POINT ( 'NONE',  ( -5.444914386472299306, 39.31328125108394289, 13.14518615778179722 ) ) ;
#17056=FACE_OUTER_BOUND ( 'NONE', #4683, .T. ) ;
#17067=CARTESIAN_POINT ( 'NONE',  ( -13.57481594606304398, 34.00507812716787726, 5.622872871577880183 ) ) ;
#17101=CARTESIAN_POINT ( 'NONE',  ( -13.14518615778179189, 36.63437500108393863, 5.444914386472304635 ) ) ;
#17117=DIRECTION ( 'NONE',  ( -0.000000000000000000, -1.000000000000000000, -0.000000000000000000 ) ) ;
#17123=CARTESIAN_POINT ( 'NONE',  ( -5.444914386472299306, 32.96328125108393436, 13.14518615778179722 ) ) ;
#17132=FACE_OUTER_BOUND ( 'NONE', #23562, .T. ) ;
#17143=CARTESIAN_POINT ( 'NONE',  ( 5.622872871577870413, 37.57695312499999574, -13.57481594606304753 ) ) ;
#17148=CARTESIAN_POINT ( 'NONE',  ( 13.14518615778179544, 38.76757812608393294, -1.609821015232357215E-15 ) ) ;
#17151=CARTESIAN_POINT ( 'NONE',  ( 13.57481594606304753, 38.27148437500000711, -5.622872871577873966 ) ) ;
#17164=CARTESIAN_POINT ( 'NONE',  ( -5.622872871577873077, 35.29492187500000000, -13.57481594606304753 ) ) ;
#17165=CARTESIAN_POINT ( 'NONE',  ( -8.049105076161786076E-16, 36.38632812608393152, -13.14518615778179544 ) ) ;
#17179=CARTESIAN_POINT ( 'NONE',  ( -13.57481594606304576, 37.03124999999999289, 0.000000000000000000 ) ) ;
#17193=LINE ( 'NONE', #6370, #25883 ) ;
#17198=DIRECTION ( 'NONE',  ( -0.000000000000000000, -1.000000000000000000, -0.000000000000000000 ) ) ;
#17199=CARTESIAN_POINT ( 'NONE',  ( -9.295050272127044266, 38.46992187608393721, 9.295050272127047819 ) ) ;
#17200=CARTESIAN_POINT ( 'NONE',  ( 13.57481594606304576, 39.90859375216787441, -1.662435489736055892E-15 ) ) ;
#17212=CARTESIAN_POINT ( 'NONE',  ( 5.622872871577878406, 34.20351562716788152, 13.57481594606304398 ) ) ;
#17218=CARTESIAN_POINT ( 'NONE',  ( 13.14518615778179900, 37.82500000108392868, -5.444914386472297529 ) ) ;
#17248=CARTESIAN_POINT ( 'NONE',  ( 9.295050272127047819, 37.67617187608393436, 9.295050272127046043 ) ) ;
#17256=DIRECTION ( 'NONE',  ( -0.000000000000000000, -1.000000000000000000, -0.000000000000000000 ) ) ;
#17284=( BOUNDED_CURVE ( )  B_SPLINE_CURVE ( 2, ( #11219, #23929, #416, #4408, #8958, #9242, #13062, #24070, #26646 ),
 .UNSPECIFIED., .F., .T. ) 
 B_SPLINE_CURVE_WITH_KNOTS ( ( 3, 2, 2, 2, 3 ),
 ( 0.1875000000000001388, 0.1979166666666667407, 0.2083333333333333703, 0.2187499999999999722, 0.2291666666666665741 ),
 .UNSPECIFIED. ) 
 CURVE ( )  GEOMETRIC_REPRESENTATION_ITEM ( )  RATIONAL_B_SPLINE_CURVE ( ( 0.9999999999999990008, 0.9238795325112877377, 1.000000000000000000, 0.9238795325112867385, 1.000000000000000000, 0.9238795325112867385, 1.000000000000000000, 0.9238795325112872936, 0.9999999999999994449 ) ) 
 REPRESENTATION_ITEM ( '' )  );
#17286=CARTESIAN_POINT ( 'NONE',  ( -8.312177448680279460E-16, 37.62656249999999858, -13.57481594606304576 ) ) ;
#17290=CARTESIAN_POINT ( 'NONE',  ( 13.14518615778179900, 37.92421875108392726, 5.444914386472293977 ) ) ;
#17302=MECHANICAL_DESIGN_GEOMETRIC_PRESENTATION_REPRESENTATION('',(#18239),#6385);
#17303=CARTESIAN_POINT ( 'NONE',  ( 9.598844408820459861, 36.53515624999999289, 9.598844408820456309 ) ) ;
#17304=CARTESIAN_POINT ( 'NONE',  ( -5.444914386472299306, 36.73359375108393010, 13.14518615778179722 ) ) ;
#17326=VERTEX_POINT ( 'NONE', #18104 ) ;
#17341=AXIS2_PLACEMENT_3D ( 'NONE', #42, #23982, #1911 ) ;
#17342=ORIENTED_EDGE ( 'NONE', *, *, #15737, .T. ) ;
#17344=CARTESIAN_POINT ( 'NONE',  ( -13.14518615778179544, 35.98945312608393721, 0.000000000000000000 ) ) ;
#17345=CARTESIAN_POINT ( 'NONE',  ( 2.493653234604083739E-15, 38.91640625216786731, 13.57481594606304576 ) ) ;
#17357=SURFACE_SIDE_STYLE ('',( #21647 ) ) ;
#17359=CARTESIAN_POINT ( 'NONE',  ( 1.662435489736055892E-15, 40.99999999999999289, 13.57481594606304576 ) ) ;
#17364=CARTESIAN_POINT ( 'NONE',  ( -13.14518615778179544, 39.75976562608393294, 0.000000000000000000 ) ) ;
#17370=CARTESIAN_POINT ( 'NONE',  ( -5.622872871577920151, 35.69179687716787441, 13.57481594606300135 ) ) ;
#17378=CARTESIAN_POINT ( 'NONE',  ( 13.57481594606304753, 34.30273437500000000, -5.622872871577873966 ) ) ;
#17390=CARTESIAN_POINT ( 'NONE',  ( -13.14518615778179189, 37.42812500108393436, 5.444914386472304635 ) ) ;
#17415=ORIENTED_EDGE ( 'NONE', *, *, #9152, .F. ) ;
#17430=ORIENTED_EDGE ( 'NONE', *, *, #16124, .F. ) ;
#17433=CARTESIAN_POINT ( 'NONE',  ( 13.14518615778179544, 39.56132812608393579, -1.609821015232357215E-15 ) ) ;
#17438=CARTESIAN_POINT ( 'NONE',  ( 5.444914386472302859, 39.41250000108393436, 13.14518615778179189 ) ) ;
#17440=CARTESIAN_POINT ( 'NONE',  ( -13.57481594606304576, 39.51171875216787299, 0.000000000000000000 ) ) ;
#17445=CARTESIAN_POINT ( 'NONE',  ( -5.622872871577873077, 36.38632812499999858, 13.57481594606304753 ) ) ;
#17446=CARTESIAN_POINT ( 'NONE',  ( -9.295050272127044266, 36.68398437608392726, 9.295050272127047819 ) ) ;
#17459=CARTESIAN_POINT ( 'NONE',  ( -8.312177448680279460E-16, 36.13828125216787157, -13.57481594606304576 ) ) ;
#17477=MANIFOLD_SOLID_BREP ( 'Thread1', #3980 ) ;
#17480=EDGE_CURVE ( 'NONE', #8513, #12423, #14416, .T. ) ;
#17481=CARTESIAN_POINT ( 'NONE',  ( -5.444914386472299306, 35.34453125108393579, 13.14518615778179722 ) ) ;
#17482=CARTESIAN_POINT ( 'NONE',  ( 13.57481594606304931, 37.47773437716787726, 5.622872871577869525 ) ) ;
#17493=CARTESIAN_POINT ( 'NONE',  ( 2.493653234604083739E-15, 34.15390625216787157, 13.57481594606304576 ) ) ;
#17494=PRESENTATION_STYLE_ASSIGNMENT (( #22071 ) ) ;
#17496=( BOUNDED_CURVE ( )  B_SPLINE_CURVE ( 2, ( #8680, #17370, #15213, #11082, #16074, #20086, #5120, #11647, #13356 ),
 .UNSPECIFIED., .F., .F. ) 
 B_SPLINE_CURVE_WITH_KNOTS ( ( 3, 2, 2, 2, 3 ),
 ( 0.4791666666666667962, 0.4895833333333333703, 0.5000000000000000000, 0.5104166666666665186, 0.5208333333333332593 ),
 .UNSPECIFIED. ) 
 CURVE ( )  GEOMETRIC_REPRESENTATION_ITEM ( )  RATIONAL_B_SPLINE_CURVE ( ( 0.9999999999999992228, 0.9238795325112875156, 1.000000000000000000, 0.9238795325112867385, 1.000000000000000000, 0.9238795325112867385, 1.000000000000000000, 0.9238795325112875156, 0.9999999999999992228 ) ) 
 REPRESENTATION_ITEM ( '' )  );
#17502=CARTESIAN_POINT ( 'NONE',  ( -5.444914386472299306, 35.93984375108392726, 13.14518615778179722 ) ) ;
#17532=CARTESIAN_POINT ( 'NONE',  ( -13.14518615778179544, 34.99726562608393721, 0.000000000000000000 ) ) ;
#17533=CARTESIAN_POINT ( 'NONE',  ( 5.622872871577946796, 36.58476562716786873, 13.57481594606297115 ) ) ;
#17570=ORIENTED_EDGE ( 'NONE', *, *, #11777, .F. ) ;
#17571=VERTEX_POINT ( 'NONE', #18355 ) ;
#17572=CARTESIAN_POINT ( 'NONE',  ( -9.295050272127046043, 39.85898437608393152, -9.295050272127046043 ) ) ;
#17576=CARTESIAN_POINT ( 'NONE',  ( 5.622872871577786924, 38.07304687499999574, 13.57481594606313813 ) ) ;
#17579=CARTESIAN_POINT ( 'NONE',  ( -9.295050272127044266, 39.26367187608393294, 9.295050272127047819 ) ) ;
#17580=CARTESIAN_POINT ( 'NONE',  ( 2.493653234604083739E-15, 39.71015625216787015, 13.57481594606304576 ) ) ;
#17586=CARTESIAN_POINT ( 'NONE',  ( -5.622872871577873077, 37.97382812499999716, 13.57481594606304753 ) ) ;
#17587=CARTESIAN_POINT ( 'NONE',  ( -13.14518615778179544, 35.79101562608393294, 0.000000000000000000 ) ) ;
#17598=CARTESIAN_POINT ( 'NONE',  ( 0.000000000000000000, 30.99999999999999645, 0.000000000000000000 ) ) ;
#17602=CARTESIAN_POINT ( 'NONE',  ( -13.57481594606304753, 36.28710937716787299, -5.622872871577872189 ) ) ;
#17622=CARTESIAN_POINT ( 'NONE',  ( 13.14518615778179900, 35.64218750108393152, -5.444914386472297529 ) ) ;
#17623=CARTESIAN_POINT ( 'NONE',  ( 5.622872871577871301, 36.08867187716787583, -13.57481594606304753 ) ) ;
#17634=DIRECTION ( 'NONE',  ( 0.000000000000000000, 0.000000000000000000, -1.000000000000000000 ) ) ;
#17637=VERTEX_POINT ( 'NONE', #15912 ) ;
#17644=CARTESIAN_POINT ( 'NONE',  ( 5.444914386472297529, 36.33671875108394289, -13.14518615778179900 ) ) ;
#17675=CARTESIAN_POINT ( 'NONE',  ( 13.14518615778179722, 37.72578125108393010, 5.444914386472293977 ) ) ;
#17692=LINE ( 'NONE', #19827, #7249 ) ;
#17718=EDGE_CURVE ( 'NONE', #21855, #21025, #15491, .T. ) ;
#17723=CARTESIAN_POINT ( 'NONE',  ( -9.295050272127046043, 39.06523437608392868, -9.295050272127046043 ) ) ;
#17728=CARTESIAN_POINT ( 'NONE',  ( -9.295050272127046043, 38.27148437608393294, -9.295050272127046043 ) ) ;
#17733=ORIENTED_EDGE ( 'NONE', *, *, #7016, .F. ) ;
#17734=CARTESIAN_POINT ( 'NONE',  ( 5.622872871577871301, 35.98945312499999716, -13.57481594606304753 ) ) ;
#17735=CARTESIAN_POINT ( 'NONE',  ( 5.444914386472302859, 38.42031250108393436, 13.14518615778179189 ) ) ;
#17741=ORIENTED_EDGE ( 'NONE', *, *, #8291, .T. ) ;
#17750=CIRCLE ( 'NONE', #8657, 13.57481594606304576 ) ;
#17769=ORIENTED_EDGE ( 'NONE', *, *, #25654, .F. ) ;
#17771=CARTESIAN_POINT ( 'NONE',  ( 5.444914386472302859, 36.23750000108393721, 13.14518615778179189 ) ) ;
#17772=CARTESIAN_POINT ( 'NONE',  ( -9.598844408820458085, 37.03125000216787299, -9.598844408820458085 ) ) ;
#17785=FILL_AREA_STYLE ('',( #11208 ) ) ;
#17790=( BOUNDED_CURVE ( )  B_SPLINE_CURVE ( 2, ( #28173, #4513, #13170, #21909, #25262, #9733, #4798, #23137, #18714 ),
 .UNSPECIFIED., .F., .F. ) 
 B_SPLINE_CURVE_WITH_KNOTS ( ( 3, 2, 2, 2, 3 ),
 ( 0.8541666666666662966, 0.8645833333333331483, 0.8750000000000000000, 0.8854166666666667407, 0.8958333333333335924 ),
 .UNSPECIFIED. ) 
 CURVE ( )  GEOMETRIC_REPRESENTATION_ITEM ( )  RATIONAL_B_SPLINE_CURVE ( ( 1.000000000000002442, 0.9238795325112842960, 1.000000000000000000, 0.9238795325112867385, 1.000000000000000000, 0.9238795325112867385, 1.000000000000000000, 0.9238795325112850731, 1.000000000000001554 ) ) 
 REPRESENTATION_ITEM ( '' )  );
#17793=CARTESIAN_POINT ( 'NONE',  ( 9.295050272127046043, 36.28710937608393294, -9.295050272127046043 ) ) ;
#17818=CARTESIAN_POINT ( 'NONE',  ( 13.14518615778179544, 33.80664062608393294, -1.609821015232357215E-15 ) ) ;
#17839=EDGE_CURVE ( 'NONE', #15078, #15088, #10781, .T. ) ;
#17840=CARTESIAN_POINT ( 'NONE',  ( 0.000000000000000000, 40.99999999999999289, 0.000000000000000000 ) ) ;
#17847=VERTEX_POINT ( 'NONE', #26930 ) ;
#17849=CARTESIAN_POINT ( 'NONE',  ( 2.493653234604083739E-15, 33.36015625216786873, 13.57481594606304576 ) ) ;
#17862=CARTESIAN_POINT ( 'NONE',  ( 9.295050272127046043, 34.89804687608393863, -9.295050272127046043 ) ) ;
#17869=CARTESIAN_POINT ( 'NONE',  ( 9.295050272127047819, 37.08085937608393579, 9.295050272127046043 ) ) ;
#17874=CARTESIAN_POINT ( 'NONE',  ( -9.598844408820454532, 33.95546874999999432, 9.598844408820459861 ) ) ;
#17875=CARTESIAN_POINT ( 'NONE',  ( -13.14518615778179189, 34.25312500108393010, 5.444914386472304635 ) ) ;
#17889=CARTESIAN_POINT ( 'NONE',  ( 5.622872871578008080, 36.78320312499999289, -13.57481594606290898 ) ) ;
#17903=CARTESIAN_POINT ( 'NONE',  ( 13.57481594606304753, 35.19570312716787441, -5.622872871577873966 ) ) ;
#17910=CARTESIAN_POINT ( 'NONE',  ( 9.295050272127047819, 37.87460937608393863, 9.295050272127046043 ) ) ;
#17911=CARTESIAN_POINT ( 'NONE',  ( 2.493653234604083739E-15, 38.12265625216787157, 13.57481594606304576 ) ) ;
#17915=CARTESIAN_POINT ( 'NONE',  ( 3.878385297391210518, 32.03609435653363136, -13.57481594606304576 ) ) ;
#17922=CARTESIAN_POINT ( 'NONE',  ( -13.57481594606304576, 31.57421875216786944, 0.000000000000000000 ) ) ;
#17931=CARTESIAN_POINT ( 'NONE',  ( -13.14518615778179900, 34.94765625108392726, -5.444914386472297529 ) ) ;
#17960=CARTESIAN_POINT ( 'NONE',  ( -9.295050272127046043, 31.72304687608393081, -9.295050272127046043 ) ) ;
#18002=CARTESIAN_POINT ( 'NONE',  ( 9.295050272127046043, 36.48554687608393721, -9.295050272127046043 ) ) ;
#18007=CARTESIAN_POINT ( 'NONE',  ( -13.14518615778179189, 33.65781250108393152, 5.444914386472304635 ) ) ;
#18013=CARTESIAN_POINT ( 'NONE',  ( -8.312177448680279460E-16, 34.45156249999999432, -13.57481594606304576 ) ) ;
#18014=CARTESIAN_POINT ( 'NONE',  ( 13.14518615778179900, 33.06250000108393294, -5.444914386472297529 ) ) ;
#18017=CARTESIAN_POINT ( 'NONE',  ( 1.662435489736055892E-15, 30.99999999999999645, 13.57481594606304576 ) ) ;
#18023=DIRECTION ( 'NONE',  ( 0.000000000000000000, 1.000000000000000000, 0.000000000000000000 ) ) ;
#18034=EDGE_CURVE ( 'NONE', #7953, #2000, #10902, .T. ) ;
#18046=CARTESIAN_POINT ( 'NONE',  ( -13.57481594606304753, 40.25585937716787299, -5.622872871577872189 ) ) ;
#18047=( BOUNDED_CURVE ( )  B_SPLINE_CURVE ( 2, ( #23886, #28028, #6491, #12750, #17179, #23471, #6628, #6084, #4363 ),
 .UNSPECIFIED., .F., .F. ) 
 B_SPLINE_CURVE_WITH_KNOTS ( ( 3, 2, 2, 2, 3 ),
 ( 0.3958333333333331483, 0.4062499999999999445, 0.4166666666666667407, 0.4270833333333335369, 0.4375000000000003331 ),
 .UNSPECIFIED. ) 
 CURVE ( )  GEOMETRIC_REPRESENTATION_ITEM ( )  RATIONAL_B_SPLINE_CURVE ( ( 1.000000000000001110, 0.9238795325112855172, 1.000000000000000000, 0.9238795325112867385, 1.000000000000000000, 0.9238795325112867385, 1.000000000000000000, 0.9238795325112842960, 1.000000000000002442 ) ) 
 REPRESENTATION_ITEM ( '' )  );
#18048=CARTESIAN_POINT ( 'NONE',  ( -5.444914386472299306, 33.75703125108393721, 13.14518615778179722 ) ) ;
#18049=CARTESIAN_POINT ( 'NONE',  ( 13.57481594606304931, 33.50898437716787015, 5.622872871577869525 ) ) ;
#18070=CARTESIAN_POINT ( 'NONE',  ( 2.414731522848535132E-15, 36.78320312608393294, 13.14518615778179544 ) ) ;
#18074=CARTESIAN_POINT ( 'NONE',  ( 5.622872871577780707, 37.67617187716787441, -13.57481594606313990 ) ) ;
#18095=LINE ( 'NONE', #8834, #2233 ) ;
#18100=ORIENTED_EDGE ( 'NONE', *, *, #20458, .F. ) ;
#18101=CARTESIAN_POINT ( 'NONE',  ( -13.14518615778179722, 31.77265625108393365, -5.444914386472297529 ) ) ;
#18104=CARTESIAN_POINT ( 'NONE',  ( 2.493653234604083739E-15, 32.56640625216787299, 13.57481594606304576 ) ) ;
#18120=CARTESIAN_POINT ( 'NONE',  ( 7.171390501253594785, 31.30502191632583830, -11.52591802191987114 ) ) ;
#18125=( BOUNDED_CURVE ( )  B_SPLINE_CURVE ( 2, ( #24902, #17915, #18201 ),
 .UNSPECIFIED., .F., .T. ) 
 B_SPLINE_CURVE_WITH_KNOTS ( ( 3, 3 ),
 ( 0.9375000000000000000, 0.9448586968893691873 ),
 .UNSPECIFIED. ) 
 CURVE ( )  GEOMETRIC_REPRESENTATION_ITEM ( )  RATIONAL_B_SPLINE_CURVE ( ( 1.000000000000000000, 0.9462258450566536361, 0.9684275698016389100 ) ) 
 REPRESENTATION_ITEM ( '' )  );
#18138=CARTESIAN_POINT ( 'NONE',  ( -9.295050272127046043, 38.86679687608393863, -9.295050272127046043 ) ) ;
#18145=CARTESIAN_POINT ( 'NONE',  ( -13.14518615778179189, 35.24531250108393721, 5.444914386472304635 ) ) ;
#18150=CARTESIAN_POINT ( 'NONE',  ( 13.14518615778179722, 35.64218750108393863, -5.444914386472297529 ) ) ;
#18159=CARTESIAN_POINT ( 'NONE',  ( 5.622872871577878406, 32.51679687499999716, 13.57481594606304576 ) ) ;
#18160=CARTESIAN_POINT ( 'NONE',  ( -5.444914386472297529, 33.26093750108393721, -13.14518615778179900 ) ) ;
#18175=FILL_AREA_STYLE_COLOUR ( '', #19070 ) ;
#18194=CARTESIAN_POINT ( 'NONE',  ( 5.444914386472297529, 32.56640625108394005, -13.14518615778179900 ) ) ;
#18195=CARTESIAN_POINT ( 'NONE',  ( -8.312177448680279460E-16, 35.34453125216787583, -13.57481594606304576 ) ) ;
#18198=ADVANCED_FACE ( 'NONE', ( #20473 ), #952, .F. ) ;
#18201=CARTESIAN_POINT ( 'NONE',  ( 7.171391216998964424, 31.99955315621561525, -11.52591757658528948 ) ) ;
#18205=LINE ( 'NONE', #15483, #5317 ) ;
#18208=DIRECTION ( 'NONE',  ( -0.000000000000000000, -1.000000000000000000, -0.000000000000000000 ) ) ;
#18220=CARTESIAN_POINT ( 'NONE',  ( -13.14518615778179544, 32.61601562608393579, 0.000000000000000000 ) ) ;
#18224=CARTESIAN_POINT ( 'NONE',  ( 2.493653234604083739E-15, 40.40468749999999432, 13.57481594606304576 ) ) ;
#18225=CARTESIAN_POINT ( 'NONE',  ( -8.312177448680279460E-16, 35.24531249999999716, -13.57481594606304576 ) ) ;
#18231=EDGE_CURVE ( 'NONE', #8989, #19422, #20263, .T. ) ;
#18239=STYLED_ITEM ( 'NONE', ( #17494 ), #17477 ) ;
#18251=CARTESIAN_POINT ( 'NONE',  ( 5.444914386472297529, 32.36796875108393579, -13.14518615778179722 ) ) ;
#18292=CARTESIAN_POINT ( 'NONE',  ( -9.295050272127044266, 36.08867187608393579, 9.295050272127047819 ) ) ;
#18296=VERTEX_POINT ( 'NONE', #3641 ) ;
#18297=CARTESIAN_POINT ( 'NONE',  ( -8.049105076161786076E-16, 34.20351562608394147, -13.14518615778179544 ) ) ;
#18303=CARTESIAN_POINT ( 'NONE',  ( 5.622872871577871301, 34.40195312499999858, -13.57481594606304753 ) ) ;
#18304=CARTESIAN_POINT ( 'NONE',  ( -9.295050272127046043, 32.51679687608393721, -9.295050272127046043 ) ) ;
#18311=EDGE_LOOP ( 'NONE', ( #26254, #17342, #20321, #15293 ) ) ;
#18328=DIRECTION ( 'NONE',  ( -0.000000000000000000, -1.000000000000000000, -0.000000000000000000 ) ) ;
#18341=CARTESIAN_POINT ( 'NONE',  ( 13.14518615778179900, 33.16171875108393863, 5.444914386472293977 ) ) ;
#18342=CARTESIAN_POINT ( 'NONE',  ( -8.312177448680279460E-16, 32.96328125216787441, -13.57481594606304576 ) ) ;
#18345=PRODUCT_DEFINITION_SHAPE ( 'NONE', 'NONE',  #27055 ) ;
#18352=CARTESIAN_POINT ( 'NONE',  ( -5.622872871577965448, 31.72304687716787086, 13.57481594606295161 ) ) ;
#18355=CARTESIAN_POINT ( 'NONE',  ( -8.312177448680279460E-16, 36.03906250000000000, -13.57481594606304576 ) ) ;
#18361=CARTESIAN_POINT ( 'NONE',  ( -5.444914386472299306, 31.97109375108393436, 13.14518615778179722 ) ) ;
#18365=CARTESIAN_POINT ( 'NONE',  ( 13.57481594606304931, 37.47773437716787015, 5.622872871577868636 ) ) ;
#18368=EDGE_CURVE ( 'NONE', #24154, #15008, #26851, .T. ) ;
#18391=( BOUNDED_CURVE ( )  B_SPLINE_CURVE ( 2, ( #16723, #1627, #3895, #18855, #8166, #16858, #23146, #23421, #25557 ),
 .UNSPECIFIED., .F., .F. ) 
 B_SPLINE_CURVE_WITH_KNOTS ( ( 3, 2, 2, 2, 3 ),
 ( 0.8958333333333335924, 0.9062500000000002220, 0.9166666666666667407, 0.9270833333333334814, 0.9375000000000000000 ),
 .UNSPECIFIED. ) 
 CURVE ( )  GEOMETRIC_REPRESENTATION_ITEM ( )  RATIONAL_B_SPLINE_CURVE ( ( 0.9999999999999983347, 0.9238795325112884038, 1.000000000000000000, 0.9238795325112867385, 1.000000000000000000, 0.9238795325112867385, 1.000000000000000000, 0.9238795325112867385, 1.000000000000000000 ) ) 
 REPRESENTATION_ITEM ( '' )  );
#18392=CARTESIAN_POINT ( 'NONE',  ( 13.14518615778179544, 32.21914062608393436, -1.609821015232357215E-15 ) ) ;
#18435=CARTESIAN_POINT ( 'NONE',  ( 5.444914386472297529, 37.32890625108393579, -13.14518615778179900 ) ) ;
#18444=CARTESIAN_POINT ( 'NONE',  ( 5.444914386472302859, 36.23750000108393721, 13.14518615778179189 ) ) ;
#18450=CARTESIAN_POINT ( 'NONE',  ( 2.493653234604083739E-15, 34.05468749999999289, 13.57481594606304576 ) ) ;
#18451=CARTESIAN_POINT ( 'NONE',  ( 9.295050272127047819, 34.50117187608393010, 9.295050272127046043 ) ) ;
#18453=LINE ( 'NONE', #27811, #26143 ) ;
#18454=CARTESIAN_POINT ( 'NONE',  ( 7.020078988959679300, 31.47038648902007907, -11.28272846253492112 ) ) ;
#18456=CARTESIAN_POINT ( 'NONE',  ( -8.312177448680279460E-16, 32.96328125216787441, -13.57481594606304576 ) ) ;
#18484=CARTESIAN_POINT ( 'NONE',  ( -13.14518615778179544, 32.81445312608393294, 0.000000000000000000 ) ) ;
#18485=CARTESIAN_POINT ( 'NONE',  ( -13.57481594606304576, 34.79882812716787299, 5.622872871577880183 ) ) ;
#18506=CARTESIAN_POINT ( 'NONE',  ( -13.14518615778179900, 32.56640625108394005, -5.444914386472297529 ) ) ;
#18515=CYLINDRICAL_SURFACE ( 'NONE', #18908, 13.57481594606304576 ) ;
#18545=DIRECTION ( 'NONE',  ( 0.000000000000000000, 1.000000000000000000, 0.000000000000000000 ) ) ;
#18554=EDGE_CURVE ( 'NONE', #12423, #27263, #8855, .T. ) ;
#18563=ADVANCED_FACE ( 'NONE', ( #2317 ), #6295, .T. ) ;
#18569=ADVANCED_FACE ( 'NONE', ( #10974 ), #4168, .F. ) ;
#18576=CARTESIAN_POINT ( 'NONE',  ( -5.444914386472297529, 33.45937500108394147, -13.14518615778179900 ) ) ;
#18581=CARTESIAN_POINT ( 'NONE',  ( 13.14518615778179722, 34.84843750108393579, -5.444914386472297529 ) ) ;
#18603=( BOUNDED_CURVE ( )  B_SPLINE_CURVE ( 2, ( #3073, #944, #11738, #16594, #14444, #3350, #1640, #8179, #20744 ),
 .UNSPECIFIED., .F., .F. ) 
 B_SPLINE_CURVE_WITH_KNOTS ( ( 3, 2, 2, 2, 3 ),
 ( 0.8541666666666670737, 0.8645833333333337034, 0.8750000000000003331, 0.8854166666666669627, 0.8958333333333335924 ),
 .UNSPECIFIED. ) 
 CURVE ( )  GEOMETRIC_REPRESENTATION_ITEM ( )  RATIONAL_B_SPLINE_CURVE ( ( 0.9999999999999967804, 0.9238795325112899581, 1.000000000000000000, 0.9238795325112867385, 1.000000000000000000, 0.9238795325112867385, 1.000000000000000000, 0.9238795325112850731, 1.000000000000001554 ) ) 
 REPRESENTATION_ITEM ( '' )  );
#18622=CARTESIAN_POINT ( 'NONE',  ( 13.14518615778179900, 34.74921875108395142, 5.444914386472293977 ) ) ;
#18623=CARTESIAN_POINT ( 'NONE',  ( 13.57481594606304576, 35.14609375216787157, -1.662435489736055892E-15 ) ) ;
#18646=CARTESIAN_POINT ( 'NONE',  ( -5.444914386472297529, 31.67343750108393863, -13.14518615778179900 ) ) ;
#18702=CARTESIAN_POINT ( 'NONE',  ( 13.14518615778179722, 39.31328125108392868, 5.444914386472293977 ) ) ;
#18708=CARTESIAN_POINT ( 'NONE',  ( 3.755639919285892248, 31.78804746655075419, -13.14518615778179544 ) ) ;
#18714=CARTESIAN_POINT ( 'NONE',  ( 2.493653234604083739E-15, 32.46718749999999432, 13.57481594606304576 ) ) ;
#18719=CARTESIAN_POINT ( 'NONE',  ( 2.414731522848535132E-15, 32.21914062608393436, 13.14518615778179544 ) ) ;
#18725=CARTESIAN_POINT ( 'NONE',  ( 13.14518615778179544, 32.21914062608393436, -1.609821015232357215E-15 ) ) ;
#18756=EDGE_LOOP ( 'NONE', ( #5763, #4192, #12219, #20566 ) ) ;
#18757=CARTESIAN_POINT ( 'NONE',  ( 9.598844408820456309, 39.90859374999999432, -9.598844408820458085 ) ) ;
#18758=CARTESIAN_POINT ( 'NONE',  ( -5.444914386472299306, 39.90859375108393436, 13.14518615778179722 ) ) ;
#18766=CYLINDRICAL_SURFACE ( 'NONE', #26718, 13.57481594606304576 ) ;
#18774=CARTESIAN_POINT ( 'NONE',  ( -8.312177448680279460E-16, 32.16953125216787157, -13.57481594606304576 ) ) ;
#18793=CARTESIAN_POINT ( 'NONE',  ( -9.295050272127046043, 40.65273437608393436, -9.295050272127046043 ) ) ;
#18794=CARTESIAN_POINT ( 'NONE',  ( 5.622872871577871301, 39.26367187716787299, -13.57481594606304753 ) ) ;
#18805=LINE ( 'NONE', #10092, #15565 ) ;
#18814=CARTESIAN_POINT ( 'NONE',  ( 13.57481594606304753, 35.89023437499999858, -5.622872871577873966 ) ) ;
#18832=CARTESIAN_POINT ( 'NONE',  ( -8.312177448680279460E-16, 39.31328125216787583, -13.57481594606304576 ) ) ;
#18835=CARTESIAN_POINT ( 'NONE',  ( 5.444914386472297529, 38.71796875108393721, -13.14518615778179722 ) ) ;
#18843=CARTESIAN_POINT ( 'NONE',  ( -13.14518615778179544, 32.02070312608393010, 0.000000000000000000 ) ) ;
#18850=CARTESIAN_POINT ( 'NONE',  ( -13.14518615778179544, 32.81445312608393294, 0.000000000000000000 ) ) ;
#18855=CARTESIAN_POINT ( 'NONE',  ( -13.57481594606304398, 32.31835937499999289, 5.622872871577880183 ) ) ;
#18884=CARTESIAN_POINT ( 'NONE',  ( -8.049105076161786076E-16, 31.82226562608393650, -13.14518615778179544 ) ) ;
#18885=CARTESIAN_POINT ( 'NONE',  ( -9.295050272127046043, 40.45429687608393721, -9.295050272127046043 ) ) ;
#18908=AXIS2_PLACEMENT_3D ( 'NONE', #14219, #13651, #9383 ) ;
#18927=CARTESIAN_POINT ( 'NONE',  ( -13.14518615778179900, 39.11484375108394573, -5.444914386472297529 ) ) ;
#18947=CARTESIAN_POINT ( 'NONE',  ( 9.598844408820456309, 35.93984374999999432, -9.598844408820458085 ) ) ;
#18964=CIRCLE ( 'NONE', #20361, 15.57481594606304576 ) ;
#18971=CARTESIAN_POINT ( 'NONE',  ( -13.14518615778179189, 39.80937500108393579, 5.444914386472304635 ) ) ;
#18981=CARTESIAN_POINT ( 'NONE',  ( -9.295050272127044266, 33.70742187608393436, 9.295050272127047819 ) ) ;
#18988=CARTESIAN_POINT ( 'NONE',  ( -13.14518615778179722, 31.97109375108393792, -5.444914386472297529 ) ) ;
#18989=EDGE_CURVE ( 'NONE', #19422, #16728, #27468, .T. ) ;
#19011=FACE_OUTER_BOUND ( 'NONE', #9718, .T. ) ;
#19021=CARTESIAN_POINT ( 'NONE',  ( -5.622872871577873077, 40.85117187499999147, -13.57481594606304753 ) ) ;
#19022=CARTESIAN_POINT ( 'NONE',  ( 5.444914386472297529, 39.51171875108392584, -13.14518615778179900 ) ) ;
#19070=COLOUR_RGB ( '', 0.72549020, 0.75294118, 0.79215686) ;
#19084=CARTESIAN_POINT ( 'NONE',  ( 13.14518615778179544, 39.36289062608393152, -1.609821015232357215E-15 ) ) ;
#19093=VECTOR ( 'NONE', #4522, 1000.000000000000000 ) ;
#19114=CARTESIAN_POINT ( 'NONE',  ( -9.295050272127044266, 39.85898437608393152, 9.295050272127047819 ) ) ;
#19125=CARTESIAN_POINT ( 'NONE',  ( -13.14518615778179189, 32.07031250108393294, 5.444914386472304635 ) ) ;
#19130=ADVANCED_FACE ( 'NONE', ( #15968 ), #20831, .F. ) ;
#19143=CARTESIAN_POINT ( 'NONE',  ( 13.57481594606304753, 35.09648437499999574, -5.622872871577873966 ) ) ;
#19151=CARTESIAN_POINT ( 'NONE',  ( 2.493653234604083739E-15, 37.22968749999999716, 13.57481594606304576 ) ) ;
#19156=CARTESIAN_POINT ( 'NONE',  ( -9.295050272127044266, 32.71523437608393436, 9.295050272127047819 ) ) ;
#19169=CARTESIAN_POINT ( 'NONE',  ( -13.57481594606304576, 40.25585937499999289, 5.622872871577880183 ) ) ;
#19170=CARTESIAN_POINT ( 'NONE',  ( 5.622872871577878406, 31.82226562716787654, 13.57481594606304576 ) ) ;
#19185=DIRECTION ( 'NONE',  ( -0.000000000000000000, -1.000000000000000000, -0.000000000000000000 ) ) ;
#19207=CARTESIAN_POINT ( 'NONE',  ( -5.444914386472299306, 40.10703125108393152, 13.14518615778179722 ) ) ;
#19208=CARTESIAN_POINT ( 'NONE',  ( -5.622872871577873077, 39.66054687716786731, 13.57481594606304753 ) ) ;
#19213=ORIENTED_EDGE ( 'NONE', *, *, #6344, .T. ) ;
#19219=AXIS2_PLACEMENT_3D ( 'NONE', #20499, #19922, #15486 ) ;
#19226=CARTESIAN_POINT ( 'NONE',  ( 13.14518615778179544, 40.15664062608393436, -1.609821015232357215E-15 ) ) ;
#19229=CARTESIAN_POINT ( 'NONE',  ( 5.622872871577694553, 35.69179687499999432, 13.57481594606322695 ) ) ;
#19254=CARTESIAN_POINT ( 'NONE',  ( 13.14518615778179722, 36.13828125108393152, 5.444914386472293977 ) ) ;
#19267=CARTESIAN_POINT ( 'NONE',  ( 2.493653234604083739E-15, 38.12265625216787157, 13.57481594606304576 ) ) ;
#19277=CARTESIAN_POINT ( 'NONE',  ( -8.049105076161786076E-16, 32.61601562608393579, -13.14518615778179544 ) ) ;
#19281=CARTESIAN_POINT ( 'NONE',  ( -9.598844408820458085, 37.03125000216787299, -9.598844408820458085 ) ) ;
#19285=CARTESIAN_POINT ( 'NONE',  ( 2.493653234604083739E-15, 39.61093749999999147, 13.57481594606304576 ) ) ;
#19287=VECTOR ( 'NONE', #15342, 1000.000000000000000 ) ;
#19290=DIRECTION ( 'NONE',  ( -0.000000000000000000, -1.000000000000000000, -0.000000000000000000 ) ) ;
#19296=ORIENTED_EDGE ( 'NONE', *, *, #25878, .T. ) ;
#19298=CARTESIAN_POINT ( 'NONE',  ( -5.444914386472299306, 38.51953125108393294, 13.14518615778179722 ) ) ;
#19301=CARTESIAN_POINT ( 'NONE',  ( 5.622872871577780707, 38.37070312499999858, -13.57481594606313990 ) ) ;
#19304=CARTESIAN_POINT ( 'NONE',  ( -13.14518615778179544, 40.75195312608393294, 0.000000000000000000 ) ) ;
#19310=CARTESIAN_POINT ( 'NONE',  ( 13.57481594606304576, 36.63437499999999858, -1.662435489736055892E-15 ) ) ;
#19311=CARTESIAN_POINT ( 'NONE',  ( 2.414731522848535132E-15, 36.78320312608393294, 13.14518615778179544 ) ) ;
#19343=FACE_OUTER_BOUND ( 'NONE', #2917, .T. ) ;
#19345=CARTESIAN_POINT ( 'NONE',  ( -13.14518615778179900, 40.70234375108393721, -5.444914386472297529 ) ) ;
#19356=CARTESIAN_POINT ( 'NONE',  ( 0.000000000000000000, 40.99999999999999289, 0.000000000000000000 ) ) ;
#19363=CARTESIAN_POINT ( 'NONE',  ( -8.049105076161786076E-16, 37.97382812608393721, -13.14518615778179544 ) ) ;
#19389=CARTESIAN_POINT ( 'NONE',  ( -9.295050272127044266, 35.89023437608393152, 9.295050272127047819 ) ) ;
#19404=DIRECTION ( 'NONE',  ( -0.000000000000000000, -1.000000000000000000, -0.000000000000000000 ) ) ;
#19413=FACE_OUTER_BOUND ( 'NONE', #11649, .T. ) ;
#19420=AXIS2_PLACEMENT_3D ( 'NONE', #14972, #19404, #23691 ) ;
#19421=DIRECTION ( 'NONE',  ( -0.000000000000000000, -1.000000000000000000, -0.000000000000000000 ) ) ;
#19422=VERTEX_POINT ( 'NONE', #23793 ) ;
#19424=CARTESIAN_POINT ( 'NONE',  ( 9.598844408820456309, 33.65781250216787157, -9.598844408820458085 ) ) ;
#19435=CARTESIAN_POINT ( 'NONE',  ( 13.14518615778179900, 39.51171875108392584, 5.444914386472293977 ) ) ;
#19449=CARTESIAN_POINT ( 'NONE',  ( 5.622872871577871301, 36.78320312499999289, -13.57481594606304753 ) ) ;
#19450=CARTESIAN_POINT ( 'NONE',  ( -13.14518615778179900, 35.74140625108393721, -5.444914386472297529 ) ) ;
#19461=CARTESIAN_POINT ( 'NONE',  ( 0.000000000000000000, 40.99999999999999289, 0.000000000000000000 ) ) ;
#19465=CARTESIAN_POINT ( 'NONE',  ( -5.622872871577964560, 34.50117187499998295, -13.57481594606295339 ) ) ;
#19467=CARTESIAN_POINT ( 'NONE',  ( -5.622872871577736298, 36.18789062716787441, -13.57481594606318254 ) ) ;
#19479=ORIENTED_EDGE ( 'NONE', *, *, #19944, .T. ) ;
#19486=CARTESIAN_POINT ( 'NONE',  ( 0.000000000000000000, 40.99999999999999289, -13.57481594606304576 ) ) ;
#19487=CARTESIAN_POINT ( 'NONE',  ( 9.295050272127047819, 36.28710937608393294, 9.295050272127046043 ) ) ;
#19488=CARTESIAN_POINT ( 'NONE',  ( -9.598844408820458085, 37.82500000216787583, -9.598844408820458085 ) ) ;
#19498=CARTESIAN_POINT ( 'NONE',  ( -13.57481594606304753, 38.56914062499999574, -5.622872871577872189 ) ) ;
#19507=CARTESIAN_POINT ( 'NONE',  ( -13.14518615778179900, 39.71015625108393010, -5.444914386472297529 ) ) ;
#19523=EDGE_LOOP ( 'NONE', ( #22738, #22410, #13372, #17733 ) ) ;
#19533=CARTESIAN_POINT ( 'NONE',  ( -8.049105076161786076E-16, 36.38632812608393152, -13.14518615778179544 ) ) ;
#19537=ORIENTED_EDGE ( 'NONE', *, *, #3913, .F. ) ;
#19549=DIRECTION ( 'NONE',  ( 0.000000000000000000, 0.000000000000000000, -1.000000000000000000 ) ) ;
#19556=DIRECTION ( 'NONE',  ( -0.000000000000000000, -1.000000000000000000, -0.000000000000000000 ) ) ;
#19558=ORIENTED_EDGE ( 'NONE', *, *, #1871, .T. ) ;
#19576=CARTESIAN_POINT ( 'NONE',  ( -13.14518615778179900, 39.90859375108394147, -5.444914386472297529 ) ) ;
#19582=CARTESIAN_POINT ( 'NONE',  ( -13.14518615778179544, 36.78320312608393294, 0.000000000000000000 ) ) ;
#19583=CARTESIAN_POINT ( 'NONE',  ( -13.57481594606304398, 39.56132812716787583, 5.622872871577880183 ) ) ;
#19588=VERTEX_POINT ( 'NONE', #8964 ) ;
#19589=CARTESIAN_POINT ( 'NONE',  ( -9.598844408820458085, 37.72578124999999005, -9.598844408820458085 ) ) ;
#19590=CARTESIAN_POINT ( 'NONE',  ( 13.14518615778179544, 38.56914062608393579, -1.609821015232357215E-15 ) ) ;
#19626=CARTESIAN_POINT ( 'NONE',  ( -9.295050272127046043, 37.47773437608393010, -9.295050272127046043 ) ) ;
#19627=CARTESIAN_POINT ( 'NONE',  ( 2.493653234604083739E-15, 36.53515625216787299, 13.57481594606304576 ) ) ;
#19628=( BOUNDED_CURVE ( )  B_SPLINE_CURVE ( 2, ( #6783, #26174, #15468, #4378, #12895, #2101, #4660, #13322, #2523 ),
 .UNSPECIFIED., .F., .F. ) 
 B_SPLINE_CURVE_WITH_KNOTS ( ( 3, 2, 2, 2, 3 ),
 ( 0.1458333333333336757, 0.1562500000000002776, 0.1666666666666669072, 0.1770833333333335369, 0.1875000000000001388 ),
 .UNSPECIFIED. ) 
 CURVE ( )  GEOMETRIC_REPRESENTATION_ITEM ( )  RATIONAL_B_SPLINE_CURVE ( ( 0.9999999999999975575, 0.9238795325112891810, 1.000000000000000000, 0.9238795325112867385, 1.000000000000000000, 0.9238795325112867385, 1.000000000000000000, 0.9238795325112857393, 1.000000000000001110 ) ) 
 REPRESENTATION_ITEM ( '' )  );
#19636=CARTESIAN_POINT ( 'NONE',  ( -5.622872871577964560, 33.80664062716787299, -13.57481594606295339 ) ) ;
#19644=CARTESIAN_POINT ( 'NONE',  ( 9.295050272127047819, 36.08867187608392868, 9.295050272127046043 ) ) ;
#19673=CARTESIAN_POINT ( 'NONE',  ( 13.14518615778179722, 36.93203125108394147, 5.444914386472293977 ) ) ;
#19694=ADVANCED_FACE ( 'NONE', ( #27076 ), #18515, .F. ) ;
#19714=CARTESIAN_POINT ( 'NONE',  ( -13.14518615778179189, 40.00781250108393294, 5.444914386472304635 ) ) ;
#19719=CARTESIAN_POINT ( 'NONE',  ( 13.14518615778179722, 37.22968750108394431, -5.444914386472297529 ) ) ;
#19724=ORIENTED_EDGE ( 'NONE', *, *, #14702, .F. ) ;
#19726=CARTESIAN_POINT ( 'NONE',  ( 13.57481594606304576, 37.42812499999999432, -1.662435489736055892E-15 ) ) ;
#19727=CARTESIAN_POINT ( 'NONE',  ( -13.14518615778179544, 38.17226562608393436, 0.000000000000000000 ) ) ;
#19746=VERTEX_POINT ( 'NONE', #12351 ) ;
#19762=CARTESIAN_POINT ( 'NONE',  ( 2.493653234604083739E-15, 31.77265625216787370, 13.57481594606304576 ) ) ;
#19763=CARTESIAN_POINT ( 'NONE',  ( -13.14518615778179189, 38.42031250108393436, 5.444914386472304635 ) ) ;
#19764=CARTESIAN_POINT ( 'NONE',  ( 5.622872871577871301, 36.88242187716787157, -13.57481594606304753 ) ) ;
#19776=CARTESIAN_POINT ( 'NONE',  ( -9.598844408820458085, 33.85625000216787583, -9.598844408820458085 ) ) ;
#19778=( NAMED_UNIT ( * ) SI_UNIT ( $, .STERADIAN. ) SOLID_ANGLE_UNIT ( ) );
#19787=CARTESIAN_POINT ( 'NONE',  ( 9.295050272127046043, 35.49335937608393010, -9.295050272127046043 ) ) ;
#19804=ADVANCED_FACE ( 'NONE', ( #240 ), #2248, .F. ) ;
#19807=EDGE_LOOP ( 'NONE', ( #10127, #6003, #21592, #12987 ) ) ;
#19817=CARTESIAN_POINT ( 'NONE',  ( 5.444914386472297529, 36.33671875108393579, -13.14518615778179722 ) ) ;
#19818=CARTESIAN_POINT ( 'NONE',  ( 2.493653234604083739E-15, 36.53515625216787299, 13.57481594606304576 ) ) ;
#19827=CARTESIAN_POINT ( 'NONE',  ( 0.000000000000000000, 40.99999999999999289, -13.57481594606304576 ) ) ;
#19856=CARTESIAN_POINT ( 'NONE',  ( 5.444914386472302859, 40.20625000108394431, 13.14518615778179189 ) ) ;
#19862=CARTESIAN_POINT ( 'NONE',  ( -5.444914386472299306, 37.72578125108394431, 13.14518615778179722 ) ) ;
#19870=CARTESIAN_POINT ( 'NONE',  ( -9.598844408820454532, 37.92421874999999432, 9.598844408820459861 ) ) ;
#19871=CARTESIAN_POINT ( 'NONE',  ( -13.14518615778179544, 37.37851562608393863, 0.000000000000000000 ) ) ;
#19872=VERTEX_POINT ( 'NONE', #13175 ) ;
#19878=SHAPE_REPRESENTATION ( 'suction cup mounting thread', ( #26844 ), #9975 ) ;
#19882=CARTESIAN_POINT ( 'NONE',  ( -8.312177448680279460E-16, 32.96328125216787441, -13.57481594606304576 ) ) ;
#19909=ORIENTED_EDGE ( 'NONE', *, *, #22744, .T. ) ;
#19910=CARTESIAN_POINT ( 'NONE',  ( -8.312177448680279460E-16, 40.10703125216787157, -13.57481594606304576 ) ) ;
#19911=CARTESIAN_POINT ( 'NONE',  ( 9.295050272127047819, 37.08085937608393579, 9.295050272127046043 ) ) ;
#19912=CARTESIAN_POINT ( 'NONE',  ( -9.598844408820454532, 36.43593750216787441, 9.598844408820459861 ) ) ;
#19922=DIRECTION ( 'NONE',  ( -0.000000000000000000, -1.000000000000000000, -0.000000000000000000 ) ) ;
#19931=CARTESIAN_POINT ( 'NONE',  ( -5.444914386472299306, 37.52734375108393294, 13.14518615778179722 ) ) ;
#19944=EDGE_CURVE ( 'NONE', #16728, #19746, #19628, .T. ) ;
#19955=PRODUCT_DEFINITION_FORMATION_WITH_SPECIFIED_SOURCE ( 'ANY', '', #20393, .NOT_KNOWN. ) ;
#19963=CARTESIAN_POINT ( 'NONE',  ( 13.14518615778179722, 33.06250000108393294, -5.444914386472297529 ) ) ;
#19970=DIRECTION ( 'NONE',  ( -0.000000000000000000, -1.000000000000000000, -0.000000000000000000 ) ) ;
#19987=CYLINDRICAL_SURFACE ( 'NONE', #11213, 13.57481594606304576 ) ;
#20008=CARTESIAN_POINT ( 'NONE',  ( 5.444914386472302859, 36.23750000108393721, 13.14518615778179189 ) ) ;
#20014=CARTESIAN_POINT ( 'NONE',  ( -13.14518615778179544, 37.57695312608393579, 0.000000000000000000 ) ) ;
#20020=CARTESIAN_POINT ( 'NONE',  ( -5.622872871577873077, 33.70742187500000142, -13.57481594606304753 ) ) ;
#20021=CARTESIAN_POINT ( 'NONE',  ( -13.14518615778179189, 33.45937500108392726, 5.444914386472304635 ) ) ;
#20025=AXIS2_PLACEMENT_3D ( 'NONE', #14287, #7606, #5900 ) ;
#20034=CARTESIAN_POINT ( 'NONE',  ( -13.57481594606304398, 34.79882812716788010, 5.622872871577880183 ) ) ;
#20056=CARTESIAN_POINT ( 'NONE',  ( 9.295050272127047819, 35.49335937608393721, 9.295050272127046043 ) ) ;
#20057=CARTESIAN_POINT ( 'NONE',  ( -9.598844408820454532, 38.02343750216788010, 9.598844408820459861 ) ) ;
#20061=AXIS2_PLACEMENT_3D ( 'NONE', #25256, #5746, #20991 ) ;
#20065=DIRECTION ( 'NONE',  ( -0.000000000000000000, -1.000000000000000000, -0.000000000000000000 ) ) ;
#20079=CARTESIAN_POINT ( 'NONE',  ( 13.14518615778179900, 35.34453125108392868, 5.444914386472293977 ) ) ;
#20086=CARTESIAN_POINT ( 'NONE',  ( -13.57481594606304753, 35.49335937716787726, -5.622872871577872189 ) ) ;
#20108=EDGE_LOOP ( 'NONE', ( #6042, #4475, #10838, #3901 ) ) ;
#20109=CARTESIAN_POINT ( 'NONE',  ( 13.14518615778179722, 32.96328125108393436, 5.444914386472293977 ) ) ;
#20127=DIRECTION ( 'NONE',  ( -0.000000000000000000, -1.000000000000000000, -0.000000000000000000 ) ) ;
#20150=CARTESIAN_POINT ( 'NONE',  ( 13.14518615778179900, 37.13046875108393863, 5.444914386472293977 ) ) ;
#20156=CARTESIAN_POINT ( 'NONE',  ( 9.295050272127046043, 38.86679687608393863, -9.295050272127046043 ) ) ;
#20161=CARTESIAN_POINT ( 'NONE',  ( 13.57481594606304753, 33.50898437499999716, -5.622872871577873077 ) ) ;
#20162=CARTESIAN_POINT ( 'NONE',  ( -9.295050272127046043, 33.31054687608393294, -9.295050272127046043 ) ) ;
#20176=CARTESIAN_POINT ( 'NONE',  ( 7.171391216998964424, 31.99955315621561525, -11.52591757658528948 ) ) ;
#20195=CARTESIAN_POINT ( 'NONE',  ( -5.444914386472299306, 32.96328125108393436, 13.14518615778179722 ) ) ;
#20196=CARTESIAN_POINT ( 'NONE',  ( 5.622872871577878406, 34.20351562716788862, 13.57481594606304576 ) ) ;
#20216=CARTESIAN_POINT ( 'NONE',  ( -5.444914386472297529, 36.43593750108392726, -13.14518615778179900 ) ) ;
#20222=EDGE_CURVE ( 'NONE', #3364, #7953, #26200, .T. ) ;
#20244=CARTESIAN_POINT ( 'NONE',  ( 9.295050272127047819, 32.91367187608393152, 9.295050272127046043 ) ) ;
#20249=FACE_OUTER_BOUND ( 'NONE', #12401, .T. ) ;
#20263=( BOUNDED_CURVE ( )  B_SPLINE_CURVE ( 2, ( #10033, #16458, #10304, #5643, #25438, #27444, #14723, #27724, #23441 ),
 .UNSPECIFIED., .F., .F. ) 
 B_SPLINE_CURVE_WITH_KNOTS ( ( 3, 2, 2, 2, 3 ),
 ( 0.06250000000000004163, 0.07291666666666665741, 0.08333333333333325932, 0.09374999999999987510, 0.1041666666666664909 ),
 .UNSPECIFIED. ) 
 CURVE ( )  GEOMETRIC_REPRESENTATION_ITEM ( )  RATIONAL_B_SPLINE_CURVE ( ( 0.9999999999999996669, 0.9238795325112870716, 1.000000000000000000, 0.9238795325112867385, 1.000000000000000000, 0.9238795325112867385, 1.000000000000000000, 0.9238795325112880708, 0.9999999999999986677 ) ) 
 REPRESENTATION_ITEM ( '' )  );
#20286=CARTESIAN_POINT ( 'NONE',  ( 9.295050272127046043, 35.69179687608394147, -9.295050272127046043 ) ) ;
#20294=CARTESIAN_POINT ( 'NONE',  ( 13.14518615778179544, 33.21132812608393436, -1.609821015232357215E-15 ) ) ;
#20300=ORIENTED_EDGE ( 'NONE', *, *, #25878, .F. ) ;
#20301=CARTESIAN_POINT ( 'NONE',  ( 13.57481594606304931, 33.40976562499999858, 5.622872871577869525 ) ) ;
#20302=CARTESIAN_POINT ( 'NONE',  ( 13.14518615778179900, 35.44375000108393436, -5.444914386472297529 ) ) ;
#20308=ORIENTED_EDGE ( 'NONE', *, *, #22404, .F. ) ;
#20320=AXIS2_PLACEMENT_3D ( 'NONE', #1912, #19421, #24262 ) ;
#20321=ORIENTED_EDGE ( 'NONE', *, *, #13660, .F. ) ;
#20339=CARTESIAN_POINT ( 'NONE',  ( -5.622872871577767384, 40.15664062716787441, -13.57481594606315412 ) ) ;
#20340=CARTESIAN_POINT ( 'NONE',  ( 13.14518615778179900, 33.26093750108393721, -5.444914386472297529 ) ) ;
#20341=CARTESIAN_POINT ( 'NONE',  ( -5.622872871577873077, 33.01289062716787726, -13.57481594606304753 ) ) ;
#20361=AXIS2_PLACEMENT_3D ( 'NONE', #3008, #18545, #14387 ) ;
#20363=CARTESIAN_POINT ( 'NONE',  ( 5.444914386472297529, 32.36796875108393579, -13.14518615778179900 ) ) ;
#20391=( BOUNDED_CURVE ( )  B_SPLINE_CURVE ( 2, ( #11347, #18352, #548, #9229, #17922, #7363, #22639, #13912, #3107 ),
 .UNSPECIFIED., .F., .F. ) 
 B_SPLINE_CURVE_WITH_KNOTS ( ( 3, 2, 2, 2, 3 ),
 ( 0.8958333333333335924, 0.9062500000000002220, 0.9166666666666667407, 0.9270833333333334814, 0.9375000000000000000 ),
 .UNSPECIFIED. ) 
 CURVE ( )  GEOMETRIC_REPRESENTATION_ITEM ( )  RATIONAL_B_SPLINE_CURVE ( ( 0.9999999999999983347, 0.9238795325112884038, 1.000000000000000000, 0.9238795325112867385, 1.000000000000000000, 0.9238795325112867385, 1.000000000000000000, 0.9238795325112867385, 1.000000000000000000 ) ) 
 REPRESENTATION_ITEM ( '' )  );
#20392=CARTESIAN_POINT ( 'NONE',  ( -13.14518615778179722, 33.36015625108393579, -5.444914386472297529 ) ) ;
#20393=PRODUCT ( 'suction cup mounting thread', 'suction cup mounting thread', '', ( #5718 ) ) ;
#20394=CARTESIAN_POINT ( 'NONE',  ( 13.57481594606304753, 36.78320312716788010, -5.622872871577873966 ) ) ;
#20401=CARTESIAN_POINT ( 'NONE',  ( 13.57481594606304753, 35.98945312716787015, -5.622872871577873966 ) ) ;
#20410=ORIENTED_EDGE ( 'NONE', *, *, #25719, .T. ) ;
#20419=EDGE_CURVE ( 'NONE', #5311, #19746, #4484, .T. ) ;
#20420=ORIENTED_EDGE ( 'NONE', *, *, #21282, .F. ) ;
#20436=CARTESIAN_POINT ( 'NONE',  ( -9.295050272127044266, 34.50117187608393721, 9.295050272127047819 ) ) ;
#20442=CARTESIAN_POINT ( 'NONE',  ( 9.295050272127046043, 34.89804687608393863, -9.295050272127046043 ) ) ;
#20449=CARTESIAN_POINT ( 'NONE',  ( -13.57481594606304753, 34.60039062499999574, -5.622872871577873077 ) ) ;
#20450=CARTESIAN_POINT ( 'NONE',  ( -5.444914386472297529, 32.46718750108393436, -13.14518615778179900 ) ) ;
#20458=EDGE_CURVE ( 'NONE', #15008, #10223, #6885, .T. ) ;
#20473=FACE_OUTER_BOUND ( 'NONE', #10366, .T. ) ;
#20484=ORIENTED_EDGE ( 'NONE', *, *, #16124, .T. ) ;
#20486=CARTESIAN_POINT ( 'NONE',  ( 9.295050272127047819, 33.90585937608393863, 9.295050272127046043 ) ) ;
#20487=CARTESIAN_POINT ( 'NONE',  ( -13.57481594606304576, 34.74921875216787726, 0.000000000000000000 ) ) ;
#20499=CARTESIAN_POINT ( 'NONE',  ( 0.000000000000000000, 40.99999999999999289, 0.000000000000000000 ) ) ;
#20506=CARTESIAN_POINT ( 'NONE',  ( -9.598844408820454532, 33.16171874999999858, 9.598844408820459861 ) ) ;
#20508=CARTESIAN_POINT ( 'NONE',  ( 13.14518615778179544, 33.01289062608393010, -1.609821015232357215E-15 ) ) ;
#20512=CARTESIAN_POINT ( 'NONE',  ( 13.57481594606304753, 37.57695312716787583, -5.622872871577873966 ) ) ;
#20538=CARTESIAN_POINT ( 'NONE',  ( 9.295050272127046043, 33.90585937608393152, -9.295050272127046043 ) ) ;
#20559=CARTESIAN_POINT ( 'NONE',  ( 9.598844408820459861, 39.80937500216786873, 9.598844408820456309 ) ) ;
#20563=( BOUNDED_CURVE ( )  B_SPLINE_CURVE ( 2, ( #3566, #10370, #25220 ),
 .UNSPECIFIED., .F., .F. ) 
 B_SPLINE_CURVE_WITH_KNOTS ( ( 3, 3 ),
 ( 0.9375000000000000000, 0.9448586960708869054 ),
 .UNSPECIFIED. ) 
 CURVE ( )  GEOMETRIC_REPRESENTATION_ITEM ( )  RATIONAL_B_SPLINE_CURVE ( ( 1.000000000000000000, 0.9462258510377660192, 0.9684275648627984623 ) ) 
 REPRESENTATION_ITEM ( '' )  );
#20566=ORIENTED_EDGE ( 'NONE', *, *, #9667, .T. ) ;
#20576=CARTESIAN_POINT ( 'NONE',  ( -8.312177448680279460E-16, 38.51953125216787299, -13.57481594606304576 ) ) ;
#20577=CARTESIAN_POINT ( 'NONE',  ( 13.14518615778179544, 35.59257812608393579, -1.609821015232357215E-15 ) ) ;
#20583=CARTESIAN_POINT ( 'NONE',  ( -13.14518615778179722, 33.55859375108393294, -5.444914386472297529 ) ) ;
#20589=CARTESIAN_POINT ( 'NONE',  ( -5.622872871577873077, 32.91367187499999858, -13.57481594606304753 ) ) ;
#20590=CARTESIAN_POINT ( 'NONE',  ( -9.295050272127044266, 35.09648437608392868, 9.295050272127047819 ) ) ;
#20603=CARTESIAN_POINT ( 'NONE',  ( -8.312177448680279460E-16, 34.55078125216787299, -13.57481594606304576 ) ) ;
#20608=VERTEX_POINT ( 'NONE', #6747 ) ;
#20624=CARTESIAN_POINT ( 'NONE',  ( 9.295050272127046043, 33.31054687608394005, -9.295050272127046043 ) ) ;
#20625=CARTESIAN_POINT ( 'NONE',  ( -8.312177448680279460E-16, 33.75703125216787726, -13.57481594606304576 ) ) ;
#20626=APPLICATION_CONTEXT ( 'automotive_design' ) ;
#20648=CARTESIAN_POINT ( 'NONE',  ( -13.14518615778179900, 31.77265625108393365, -5.444914386472297529 ) ) ;
#20655=DIRECTION ( 'NONE',  ( 0.8660254037844407060, 0.4999999999999963363, 0.000000000000000000 ) ) ;
#20656=EDGE_CURVE ( 'NONE', #19872, #17571, #14540, .T. ) ;
#20661=ORIENTED_EDGE ( 'NONE', *, *, #17718, .T. ) ;
#20699=VECTOR ( 'NONE', #19556, 1000.000000000000000 ) ;
#20718=CARTESIAN_POINT ( 'NONE',  ( -9.295050272127046043, 34.30273437608393294, -9.295050272127046043 ) ) ;
#20720=( BOUNDED_CURVE ( )  B_SPLINE_CURVE ( 2, ( #5543, #846, #20506, #3388, #989, #9657, #14067, #11924, #9798 ),
 .UNSPECIFIED., .F., .F. ) 
 B_SPLINE_CURVE_WITH_KNOTS ( ( 3, 2, 2, 2, 3 ),
 ( 0.8124999999999998890, 0.8229166666666665186, 0.8333333333333331483, 0.8437499999999997780, 0.8541666666666662966 ),
 .UNSPECIFIED. ) 
 CURVE ( )  GEOMETRIC_REPRESENTATION_ITEM ( )  RATIONAL_B_SPLINE_CURVE ( ( 1.000000000000000888, 0.9238795325112859613, 1.000000000000000000, 0.9238795325112867385, 1.000000000000000000, 0.9238795325112867385, 1.000000000000000000, 0.9238795325112891810, 0.9999999999999975575 ) ) 
 REPRESENTATION_ITEM ( '' )  );
#20725=CARTESIAN_POINT ( 'NONE',  ( -13.14518615778179722, 35.93984375108393436, -5.444914386472297529 ) ) ;
#20732=CARTESIAN_POINT ( 'NONE',  ( 6.944423797152705191, 31.55306878032414986, -11.16113333171310451 ) ) ;
#20744=CARTESIAN_POINT ( 'NONE',  ( 2.493653234604083739E-15, 31.77265625216787370, 13.57481594606304576 ) ) ;
#20760=CARTESIAN_POINT ( 'NONE',  ( -8.312177448680279460E-16, 36.93203125216787441, -13.57481594606304576 ) ) ;
#20761=CARTESIAN_POINT ( 'NONE',  ( -13.14518615778179189, 34.45156250108394147, 5.444914386472304635 ) ) ;
#20762=CARTESIAN_POINT ( 'NONE',  ( 2.493653234604083739E-15, 33.36015625216786873, 13.57481594606304576 ) ) ;
#20773=ORIENTED_EDGE ( 'NONE', *, *, #18554, .F. ) ;
#20786=CARTESIAN_POINT ( 'NONE',  ( 2.414731522848535132E-15, 32.81445312608393294, 13.14518615778179544 ) ) ;
#20803=CARTESIAN_POINT ( 'NONE',  ( 2.493653234604083739E-15, 33.36015625216786873, 13.57481594606304576 ) ) ;
#20824=CARTESIAN_POINT ( 'NONE',  ( 9.598844408820459861, 35.74140624999999716, 9.598844408820456309 ) ) ;
#20830=CARTESIAN_POINT ( 'NONE',  ( 2.493653234604083739E-15, 39.61093749999999147, 13.57481594606304576 ) ) ;
#20831=CYLINDRICAL_SURFACE ( 'NONE', #10251, 13.57481594606304576 ) ;
#20840=ORIENTED_EDGE ( 'NONE', *, *, #22765, .F. ) ;
#20855=CARTESIAN_POINT ( 'NONE',  ( -8.049105076161786076E-16, 31.82226562608393650, -13.14518615778179544 ) ) ;
#20862=CARTESIAN_POINT ( 'NONE',  ( -13.14518615778179544, 34.40195312608393152, 0.000000000000000000 ) ) ;
#20871=CARTESIAN_POINT ( 'NONE',  ( 2.493653234604083739E-15, 38.12265625216787157, 13.57481594606304576 ) ) ;
#20874=ORIENTED_EDGE ( 'NONE', *, *, #25719, .F. ) ;
#20876=DIRECTION ( 'NONE',  ( 0.000000000000000000, 0.000000000000000000, -1.000000000000000000 ) ) ;
#20894=CARTESIAN_POINT ( 'NONE',  ( 0.000000000000000000, 30.99999999999999645, 0.000000000000000000 ) ) ;
#20903=CARTESIAN_POINT ( 'NONE',  ( 5.622872871577871301, 40.75195312500000711, -13.57481594606304753 ) ) ;
#20904=CARTESIAN_POINT ( 'NONE',  ( -13.57481594606304753, 31.52460937716787370, -5.622872871577873077 ) ) ;
#20922=CARTESIAN_POINT ( 'NONE',  ( 2.493653234604083739E-15, 32.56640625216787299, 13.57481594606304576 ) ) ;
#20924=CARTESIAN_POINT ( 'NONE',  ( 9.598844408820456309, 40.70234374999999716, -9.598844408820458085 ) ) ;
#20940=CARTESIAN_POINT ( 'NONE',  ( -9.295050272127046043, 39.85898437608393152, -9.295050272127046043 ) ) ;
#20941=CARTESIAN_POINT ( 'NONE',  ( -5.622872871577873077, 39.36289062716787157, -13.57481594606304753 ) ) ;
#20949=EDGE_LOOP ( 'NONE', ( #22150, #12209, #19479, #14014 ) ) ;
#20985=CARTESIAN_POINT ( 'NONE',  ( -8.049105076161786076E-16, 38.76757812608393294, -13.14518615778179544 ) ) ;
#20991=DIRECTION ( 'NONE',  ( 0.000000000000000000, 0.000000000000000000, 1.000000000000000000 ) ) ;
#20994=CARTESIAN_POINT ( 'NONE',  ( -8.049105076161786076E-16, 32.61601562608393579, -13.14518615778179544 ) ) ;
#21018=CARTESIAN_POINT ( 'NONE',  ( -9.598844408820458085, 33.75703124999999005, -9.598844408820458085 ) ) ;
#21022=CARTESIAN_POINT ( 'NONE',  ( 7.114649318941503431, 31.93754143773660203, -11.43472154218138570 ) ) ;
#21025=VERTEX_POINT ( 'NONE', #11655 ) ;
#21037=CARTESIAN_POINT ( 'NONE',  ( -13.57481594606304398, 37.18007812716787441, 5.622872871577880183 ) ) ;
#21038=CARTESIAN_POINT ( 'NONE',  ( -5.622872871577873077, 38.46992187499999716, -13.57481594606304753 ) ) ;
#21039=CARTESIAN_POINT ( 'NONE',  ( 9.295050272127047819, 40.05742187608392868, 9.295050272127046043 ) ) ;
#21064=CARTESIAN_POINT ( 'NONE',  ( 0.000000000000000000, 40.99999999999999289, 0.000000000000000000 ) ) ;
#21075=CARTESIAN_POINT ( 'NONE',  ( -8.049105076161786076E-16, 39.75976562608394005, -13.14518615778179544 ) ) ;
#21112=CARTESIAN_POINT ( 'NONE',  ( -5.622872871577965448, 33.31054687716787299, 13.57481594606295161 ) ) ;
#21118=CARTESIAN_POINT ( 'NONE',  ( 9.295050272127047819, 38.46992187608393010, 9.295050272127046043 ) ) ;
#21128=CARTESIAN_POINT ( 'NONE',  ( -9.295050272127044266, 32.91367187608393152, 9.295050272127047819 ) ) ;
#21143=CARTESIAN_POINT ( 'NONE',  ( 2.493653234604083739E-15, 32.56640625216787299, 13.57481594606304576 ) ) ;
#21174=CARTESIAN_POINT ( 'NONE',  ( 3.755638155860017591, 31.78804748261757140, -13.14518615778179367 ) ) ;
#21175=CARTESIAN_POINT ( 'NONE',  ( -13.14518615778179900, 40.50390625108394005, -5.444914386472297529 ) ) ;
#21184=DIRECTION ( 'NONE',  ( -0.000000000000000000, -1.000000000000000000, -0.000000000000000000 ) ) ;
#21191=ADVANCED_FACE ( 'NONE', ( #27909 ), #5985, .F. ) ;
#21233=CARTESIAN_POINT ( 'NONE',  ( 9.295050272127047819, 39.26367187608393294, 9.295050272127046043 ) ) ;
#21246=ORIENTED_EDGE ( 'NONE', *, *, #12984, .T. ) ;
#21252=EDGE_LOOP ( 'NONE', ( #92, #11174, #26294, #10814 ) ) ;
#21260=CARTESIAN_POINT ( 'NONE',  ( -13.14518615778179189, 39.01562500108393294, 5.444914386472304635 ) ) ;
#21261=DIRECTION ( 'NONE',  ( -0.000000000000000000, -1.000000000000000000, -0.000000000000000000 ) ) ;
#21269=CARTESIAN_POINT ( 'NONE',  ( 13.14518615778179900, 32.46718750108393436, -5.444914386472297529 ) ) ;
#21277=CARTESIAN_POINT ( 'NONE',  ( 3.755639919285892248, 31.78804746655075775, -13.14518615778179544 ) ) ;
#21282=EDGE_CURVE ( 'NONE', #14317, #947, #18391, .T. ) ;
#21301=CARTESIAN_POINT ( 'NONE',  ( -13.14518615778179189, 34.25312500108393010, 5.444914386472304635 ) ) ;
#21306=DIRECTION ( 'NONE',  ( -0.000000000000000000, -1.000000000000000000, -0.000000000000000000 ) ) ;
#21311=EDGE_LOOP ( 'NONE', ( #6133, #12427, #14632, #1879 ) ) ;
#21312=CARTESIAN_POINT ( 'NONE',  ( -9.598844408820454532, 40.30546874999999574, 9.598844408820459861 ) ) ;
#21313=CARTESIAN_POINT ( 'NONE',  ( 13.14518615778179544, 39.36289062608393152, -1.609821015232357215E-15 ) ) ;
#21330=AXIS2_PLACEMENT_3D ( 'NONE', #26469, #15617, #10910 ) ;
#21343=DIRECTION ( 'NONE',  ( -0.000000000000000000, -1.000000000000000000, -0.000000000000000000 ) ) ;
#21357=CARTESIAN_POINT ( 'NONE',  ( 9.598844408820459861, 39.80937500216786873, 9.598844408820456309 ) ) ;
#21376=CARTESIAN_POINT ( 'NONE',  ( 5.444914386472297529, 39.51171875108392584, -13.14518615778179900 ) ) ;
#21405=CARTESIAN_POINT ( 'NONE',  ( -13.14518615778179722, 38.12265625108393863, -5.444914386472297529 ) ) ;
#21412=DIRECTION ( 'NONE',  ( 0.000000000000000000, 0.000000000000000000, -1.000000000000000000 ) ) ;
#21414=CARTESIAN_POINT ( 'NONE',  ( 5.622872871577912157, 38.17226562716787441, 13.57481594606301023 ) ) ;
#21445=CARTESIAN_POINT ( 'NONE',  ( -9.295050272127046043, 38.27148437608393294, -9.295050272127046043 ) ) ;
#21456=CARTESIAN_POINT ( 'NONE',  ( 13.57481594606304576, 40.60312499999999858, -1.662435489736055892E-15 ) ) ;
#21457=CARTESIAN_POINT ( 'NONE',  ( -13.14518615778179544, 38.96601562608393721, 0.000000000000000000 ) ) ;
#21489=CARTESIAN_POINT ( 'NONE',  ( -9.295050272127046043, 39.06523437608392868, -9.295050272127046043 ) ) ;
#21508=CARTESIAN_POINT ( 'NONE',  ( -13.14518615778179189, 38.22187500108393010, 5.444914386472304635 ) ) ;
#21514=EDGE_CURVE ( 'NONE', #34, #2000, #8885, .T. ) ;
#21524=EDGE_LOOP ( 'NONE', ( #8040, #24194, #4521, #16948 ) ) ;
#21530=VERTEX_POINT ( 'NONE', #5630 ) ;
#21537=CARTESIAN_POINT ( 'NONE',  ( -9.295050272127044266, 36.68398437608392726, 9.295050272127047819 ) ) ;
#21546=CYLINDRICAL_SURFACE ( 'NONE', #11392, 13.57481594606304576 ) ;
#21561=CARTESIAN_POINT ( 'NONE',  ( -9.295050272127046043, 32.71523437608393436, -9.295050272127046043 ) ) ;
#21566=ORIENTED_EDGE ( 'NONE', *, *, #8099, .T. ) ;
#21581=CARTESIAN_POINT ( 'NONE',  ( 13.14518615778179900, 40.40468750108393436, -5.444914386472297529 ) ) ;
#21584=CARTESIAN_POINT ( 'NONE',  ( 13.57481594606304576, 38.22187499999999716, -1.662435489736055892E-15 ) ) ;
#21592=ORIENTED_EDGE ( 'NONE', *, *, #27304, .F. ) ;
#21594=CARTESIAN_POINT ( 'NONE',  ( -13.57481594606304576, 35.44374999999999432, 0.000000000000000000 ) ) ;
#21595=CARTESIAN_POINT ( 'NONE',  ( -9.295050272127046043, 37.27929687608393294, -9.295050272127046043 ) ) ;
#21603=FACE_OUTER_BOUND ( 'NONE', #12523, .T. ) ;
#21632=CARTESIAN_POINT ( 'NONE',  ( 13.14518615778179544, 37.18007812608393436, -1.609821015232357215E-15 ) ) ;
#21633=CARTESIAN_POINT ( 'NONE',  ( -9.598844408820458085, 38.61875000216787157, -9.598844408820458085 ) ) ;
#21637=ADVANCED_FACE ( 'NONE', ( #10713 ), #6311, .F. ) ;
#21647=SURFACE_STYLE_FILL_AREA ( #17785 ) ;
#21653=CARTESIAN_POINT ( 'NONE',  ( 5.444914386472297529, 40.30546875108393579, -13.14518615778179900 ) ) ;
#21674=CARTESIAN_POINT ( 'NONE',  ( -13.57481594606304753, 33.11210937716787583, -5.622872871577872189 ) ) ;
#21682=CARTESIAN_POINT ( 'NONE',  ( 5.444914386472302859, 37.62656250108393152, 13.14518615778179189 ) ) ;
#21683=FACE_OUTER_BOUND ( 'NONE', #4377, .T. ) ;
#21691=EDGE_CURVE ( 'NONE', #26276, #21956, #18205, .T. ) ;
#21729=CARTESIAN_POINT ( 'NONE',  ( -13.14518615778179544, 39.16445312608393436, 0.000000000000000000 ) ) ;
#21731=CARTESIAN_POINT ( 'NONE',  ( 2.493653234604083739E-15, 38.02343749999999289, 13.57481594606304576 ) ) ;
#21734=CARTESIAN_POINT ( 'NONE',  ( 9.295050272127047819, 38.66835937608393436, 9.295050272127046043 ) ) ;
#21736=DIRECTION ( 'NONE',  ( -0.000000000000000000, -1.000000000000000000, -0.000000000000000000 ) ) ;
#21740=CARTESIAN_POINT ( 'NONE',  ( -13.57481594606304753, 35.39414062499999147, -5.622872871577873077 ) ) ;
#21741=CARTESIAN_POINT ( 'NONE',  ( -9.295050272127044266, 35.89023437608393152, 9.295050272127047819 ) ) ;
#21753=DIRECTION ( 'NONE',  ( 0.000000000000000000, -0.000000000000000000, 1.000000000000000000 ) ) ;
#21755=CARTESIAN_POINT ( 'NONE',  ( -13.57481594606304398, 34.69960937499999432, 5.622872871577880183 ) ) ;
#21769=CARTESIAN_POINT ( 'NONE',  ( 2.493653234604083739E-15, 37.22968749999999716, 13.57481594606304576 ) ) ;
#21776=CARTESIAN_POINT ( 'NONE',  ( -9.295050272127044266, 37.67617187608393436, 9.295050272127047819 ) ) ;
#21777=CARTESIAN_POINT ( 'NONE',  ( 13.57481594606304576, 37.52734375216787299, -1.662435489736055892E-15 ) ) ;
#21799=CARTESIAN_POINT ( 'NONE',  ( 0.000000000000000000, 40.99999999999999289, 0.000000000000000000 ) ) ;
#21816=ORIENTED_EDGE ( 'NONE', *, *, #18034, .F. ) ;
#21827=CARTESIAN_POINT ( 'NONE',  ( 13.14518615778179722, 37.82500000108392868, -5.444914386472297529 ) ) ;
#21835=AXIS2_PLACEMENT_3D ( 'NONE', #23310, #21306, #8325 ) ;
#21851=ORIENTED_EDGE ( 'NONE', *, *, #12453, .T. ) ;
#21855=VERTEX_POINT ( 'NONE', #27054 ) ;
#21857=CARTESIAN_POINT ( 'NONE',  ( 13.57481594606304753, 33.60820312716787583, -5.622872871577873966 ) ) ;
#21868=CARTESIAN_POINT ( 'NONE',  ( -9.295050272127044266, 37.67617187608393436, 9.295050272127047819 ) ) ;
#21871=CARTESIAN_POINT ( 'NONE',  ( -8.312177448680279460E-16, 38.42031249999999432, -13.57481594606304576 ) ) ;
#21875=CARTESIAN_POINT ( 'NONE',  ( -13.14518615778179722, 36.73359375108393010, -5.444914386472297529 ) ) ;
#21876=CARTESIAN_POINT ( 'NONE',  ( -8.312177448680279460E-16, 39.31328125216787583, -13.57481594606304576 ) ) ;
#21880=ADVANCED_FACE ( 'NONE', ( #1532 ), #18766, .F. ) ;
#21883=CARTESIAN_POINT ( 'NONE',  ( -13.57481594606304576, 35.49335937499999005, 5.622872871577880183 ) ) ;
#21884=CARTESIAN_POINT ( 'NONE',  ( -13.14518615778179544, 36.58476562608393579, 0.000000000000000000 ) ) ;
#21895=CARTESIAN_POINT ( 'NONE',  ( 2.493653234604083739E-15, 38.02343749999999289, 13.57481594606304576 ) ) ;
#21909=CARTESIAN_POINT ( 'NONE',  ( 13.57481594606304753, 32.71523437500000142, -5.622872871577873966 ) ) ;
#21921=CARTESIAN_POINT ( 'NONE',  ( 5.444914386472297529, 35.74140625108393721, -13.14518615778179900 ) ) ;
#21922=CARTESIAN_POINT ( 'NONE',  ( -13.57481594606304576, 38.76757812716787299, 5.622872871577880183 ) ) ;
#21931=CARTESIAN_POINT ( 'NONE',  ( 9.598844408820456309, 34.45156250216787441, -9.598844408820458085 ) ) ;
#21933=EDGE_LOOP ( 'NONE', ( #11949, #19909, #11157, #11692 ) ) ;
#21937=CARTESIAN_POINT ( 'NONE',  ( 0.000000000000000000, 40.99999999999999289, 0.000000000000000000 ) ) ;
#21939=CARTESIAN_POINT ( 'NONE',  ( 9.295050272127047819, 36.88242187608393152, 9.295050272127046043 ) ) ;
#21956=VERTEX_POINT ( 'NONE', #14330 ) ;
#21965=CARTESIAN_POINT ( 'NONE',  ( 13.14518615778179544, 36.98164062608393010, -1.609821015232357215E-15 ) ) ;
#21973=CARTESIAN_POINT ( 'NONE',  ( 2.493653234604083739E-15, 38.81718749999999574, 13.57481594606304576 ) ) ;
#21999=CARTESIAN_POINT ( 'NONE',  ( 9.598844408820456309, 37.52734375000000000, -9.598844408820458085 ) ) ;
#22003=CARTESIAN_POINT ( 'NONE',  ( 2.414731522848535132E-15, 38.56914062608393579, 13.14518615778179544 ) ) ;
#22009=CARTESIAN_POINT ( 'NONE',  ( -8.049105076161786076E-16, 37.37851562608393863, -13.14518615778179544 ) ) ;
#22011=CARTESIAN_POINT ( 'NONE',  ( 0.000000000000000000, 40.99999999999999289, -13.57481594606304576 ) ) ;
#22016=CARTESIAN_POINT ( 'NONE',  ( -9.598844408820458085, 36.13828124999999147, -9.598844408820458085 ) ) ;
#22017=CARTESIAN_POINT ( 'NONE',  ( 9.295050272127047819, 38.46992187608393010, 9.295050272127046043 ) ) ;
#22049=CARTESIAN_POINT ( 'NONE',  ( 0.000000000000000000, 40.99999999999999289, 0.000000000000000000 ) ) ;
#22053=EDGE_CURVE ( 'NONE', #138, #9928, #2157, .T. ) ;
#22056=CARTESIAN_POINT ( 'NONE',  ( -13.14518615778179189, 37.62656250108393863, 5.444914386472304635 ) ) ;
#22057=CARTESIAN_POINT ( 'NONE',  ( 5.622872871577878406, 35.79101562716787299, 13.57481594606304576 ) ) ;
#22070=ADVANCED_FACE ( 'NONE', ( #21603 ), #8765, .F. ) ;
#22071=SURFACE_STYLE_USAGE ( .BOTH. , #17357 ) ;
#22078=CARTESIAN_POINT ( 'NONE',  ( -13.14518615778179544, 34.99726562608393721, 0.000000000000000000 ) ) ;
#22081=DIRECTION ( 'NONE',  ( -0.000000000000000000, -1.000000000000000000, -0.000000000000000000 ) ) ;
#22106=CARTESIAN_POINT ( 'NONE',  ( -5.444914386472297529, 37.22968750108394431, -13.14518615778179722 ) ) ;
#22144=ORIENTED_EDGE ( 'NONE', *, *, #22680, .F. ) ;
#22145=CARTESIAN_POINT ( 'NONE',  ( -5.444914386472299306, 36.93203125108394147, 13.14518615778179722 ) ) ;
#22150=ORIENTED_EDGE ( 'NONE', *, *, #14163, .F. ) ;
#22151=CARTESIAN_POINT ( 'NONE',  ( 9.295050272127046043, 36.48554687608393721, -9.295050272127046043 ) ) ;
#22159=CARTESIAN_POINT ( 'NONE',  ( -13.57481594606304753, 36.98164062499999005, -5.622872871577873077 ) ) ;
#22160=CARTESIAN_POINT ( 'NONE',  ( -13.14518615778179900, 37.32890625108393579, -5.444914386472297529 ) ) ;
#22187=CARTESIAN_POINT ( 'NONE',  ( 9.598844408820456309, 35.24531250216787726, -9.598844408820458085 ) ) ;
#22195=CARTESIAN_POINT ( 'NONE',  ( 9.295050272127046043, 37.27929687608394005, -9.295050272127046043 ) ) ;
#22196=CARTESIAN_POINT ( 'NONE',  ( -13.57481594606304576, 38.71796875216787726, 0.000000000000000000 ) ) ;
#22209=CARTESIAN_POINT ( 'NONE',  ( 9.598844408820459861, 34.25312500216787015, 9.598844408820456309 ) ) ;
#22217=CARTESIAN_POINT ( 'NONE',  ( -9.295050272127046043, 35.69179687608393436, -9.295050272127046043 ) ) ;
#22220=CARTESIAN_POINT ( 'NONE',  ( 9.598844408820456309, 37.62656250216787157, -9.598844408820458085 ) ) ;
#22248=CARTESIAN_POINT ( 'NONE',  ( -9.295050272127046043, 33.31054687608393294, -9.295050272127046043 ) ) ;
#22274=VERTEX_POINT ( 'NONE', #19882 ) ;
#22277=ORIENTED_EDGE ( 'NONE', *, *, #10019, .F. ) ;
#22290=CARTESIAN_POINT ( 'NONE',  ( 13.14518615778179900, 35.54296875108394715, 5.444914386472293977 ) ) ;
#22296=CARTESIAN_POINT ( 'NONE',  ( -9.295050272127044266, 36.88242187608393152, 9.295050272127047819 ) ) ;
#22302=CARTESIAN_POINT ( 'NONE',  ( 13.57481594606304753, 32.71523437500000142, -5.622872871577873077 ) ) ;
#22303=CARTESIAN_POINT ( 'NONE',  ( 9.295050272127046043, 35.49335937608393010, -9.295050272127046043 ) ) ;
#22319=VECTOR ( 'NONE', #20655, 1000.000000000000227 ) ;
#22339=CARTESIAN_POINT ( 'NONE',  ( -13.14518615778179900, 33.55859375108393294, -5.444914386472297529 ) ) ;
#22340=CARTESIAN_POINT ( 'NONE',  ( -5.622872871577873077, 35.69179687716786731, 13.57481594606304753 ) ) ;
#22350=CYLINDRICAL_SURFACE ( 'NONE', #19219, 13.57481594606304576 ) ;
#22356=CARTESIAN_POINT ( 'NONE',  ( -9.295050272127046043, 34.89804687608393152, -9.295050272127046043 ) ) ;
#22386=CARTESIAN_POINT ( 'NONE',  ( 2.414731522848535132E-15, 32.02070312608393010, 13.14518615778179544 ) ) ;
#22404=EDGE_CURVE ( 'NONE', #5570, #11263, #16553, .T. ) ;
#22406=CARTESIAN_POINT ( 'NONE',  ( 2.493653234604083739E-15, 34.94765625216787441, 13.57481594606304576 ) ) ;
#22410=ORIENTED_EDGE ( 'NONE', *, *, #470, .T. ) ;
#22431=CARTESIAN_POINT ( 'NONE',  ( 13.14518615778179544, 37.18007812608393436, -1.609821015232357215E-15 ) ) ;
#22437=CARTESIAN_POINT ( 'NONE',  ( 9.295050272127046043, 33.31054687608394005, -9.295050272127046043 ) ) ;
#22445=CARTESIAN_POINT ( 'NONE',  ( 9.295050272127047819, 33.70742187608393436, 9.295050272127046043 ) ) ;
#22461=( NAMED_UNIT ( * ) PLANE_ANGLE_UNIT ( ) SI_UNIT ( $, .RADIAN. ) );
#22470=AXIS2_PLACEMENT_3D ( 'NONE', #19356, #13195, #17634 ) ;
#22480=CARTESIAN_POINT ( 'NONE',  ( -13.14518615778179900, 32.76484375108393010, -5.444914386472297529 ) ) ;
#22481=CARTESIAN_POINT ( 'NONE',  ( 13.57481594606304753, 33.60820312716787583, -5.622872871577873077 ) ) ;
#22500=CARTESIAN_POINT ( 'NONE',  ( 13.14518615778179900, 36.93203125108394147, 5.444914386472293977 ) ) ;
#22504=CARTESIAN_POINT ( 'NONE',  ( 2.493653234604083739E-15, 35.64218749999999147, 13.57481594606304576 ) ) ;
#22520=VECTOR ( 'NONE', #12489, 1000.000000000000000 ) ;
#22524=ORIENTED_EDGE ( 'NONE', *, *, #22765, .T. ) ;
#22527=ORIENTED_EDGE ( 'NONE', *, *, #20222, .F. ) ;
#22530=CARTESIAN_POINT ( 'NONE',  ( -9.295050272127046043, 32.51679687608393721, -9.295050272127046043 ) ) ;
#22550=CARTESIAN_POINT ( 'NONE',  ( 5.622872871577976994, 40.05742187716787583, -13.57481594606294095 ) ) ;
#22553=EDGE_CURVE ( 'NONE', #13728, #19422, #18805, .T. ) ;
#22574=CARTESIAN_POINT ( 'NONE',  ( 5.444914386472302859, 34.65000000108393863, 13.14518615778179189 ) ) ;
#22580=CARTESIAN_POINT ( 'NONE',  ( 13.14518615778179544, 35.59257812608393579, -1.609821015232357215E-15 ) ) ;
#22588=CARTESIAN_POINT ( 'NONE',  ( -9.598844408820454532, 34.74921874999999716, 9.598844408820459861 ) ) ;
#22589=CARTESIAN_POINT ( 'NONE',  ( -13.14518615778179189, 32.66562500108393863, 5.444914386472304635 ) ) ;
#22605=CARTESIAN_POINT ( 'NONE',  ( 6.944426393311537993, 31.75150625057403175, -11.16113171639042356 ) ) ;
#22607=FILL_AREA_STYLE ('',( #18175 ) ) ;
#22624=CARTESIAN_POINT ( 'NONE',  ( -13.14518615778179189, 35.24531250108393721, 5.444914386472304635 ) ) ;
#22625=CARTESIAN_POINT ( 'NONE',  ( -9.598844408820454532, 35.64218750216787868, 9.598844408820459861 ) ) ;
#22639=CARTESIAN_POINT ( 'NONE',  ( -9.598844408820458085, 31.47500000216787441, -9.598844408820458085 ) ) ;
#22646=CARTESIAN_POINT ( 'NONE',  ( 5.622872871577863307, 40.45429687500001137, 13.57481594606306174 ) ) ;
#22648=CARTESIAN_POINT ( 'NONE',  ( 2.414731522848535132E-15, 33.60820312608392868, 13.14518615778179544 ) ) ;
#22670=AXIS2_PLACEMENT_3D ( 'NONE', #17598, #4502, #21753 ) ;
#22676=CARTESIAN_POINT ( 'NONE',  ( -13.14518615778179722, 32.56640625108394005, -5.444914386472297529 ) ) ;
#22680=EDGE_CURVE ( 'NONE', #25384, #8015, #20563, .T. ) ;
#22684=CARTESIAN_POINT ( 'NONE',  ( -8.312177448680279460E-16, 36.13828125216787157, -13.57481594606304576 ) ) ;
#22697=CARTESIAN_POINT ( 'NONE',  ( 9.598844408820456309, 40.00781250216787299, -9.598844408820458085 ) ) ;
#22698=CYLINDRICAL_SURFACE ( 'NONE', #25240, 13.57481594606304576 ) ;
#22717=CARTESIAN_POINT ( 'NONE',  ( 13.14518615778179900, 37.22968750108393721, -5.444914386472297529 ) ) ;
#22724=CARTESIAN_POINT ( 'NONE',  ( -5.444914386472297529, 34.25312500108393721, -13.14518615778179722 ) ) ;
#22729=CARTESIAN_POINT ( 'NONE',  ( -13.57481594606304576, 33.11210937499999574, 5.622872871577880183 ) ) ;
#22730=CARTESIAN_POINT ( 'NONE',  ( -13.14518615778179900, 34.94765625108392726, -5.444914386472297529 ) ) ;
#22731=MECHANICAL_DESIGN_GEOMETRIC_PRESENTATION_REPRESENTATION('',(#6771),#9535);
#22738=ORIENTED_EDGE ( 'NONE', *, *, #8803, .F. ) ;
#22744=EDGE_CURVE ( 'NONE', #16597, #15008, #28058, .T. ) ;
#22765=EDGE_CURVE ( 'NONE', #12423, #17847, #5826, .T. ) ;
#22767=CARTESIAN_POINT ( 'NONE',  ( 5.444914386472302859, 33.85625000108393579, 13.14518615778179189 ) ) ;
#22768=CARTESIAN_POINT ( 'NONE',  ( 9.598844408820459861, 32.66562500216787157, 9.598844408820456309 ) ) ;
#22789=CARTESIAN_POINT ( 'NONE',  ( -13.14518615778179189, 32.66562500108393863, 5.444914386472304635 ) ) ;
#22791=ADVANCED_FACE ( 'NONE', ( #26193 ), #8944, .F. ) ;
#22817=CARTESIAN_POINT ( 'NONE',  ( -8.049105076161786076E-16, 34.00507812608393721, -13.14518615778179544 ) ) ;
#22856=CARTESIAN_POINT ( 'NONE',  ( 9.598844408820459861, 38.22187500216787015, 9.598844408820456309 ) ) ;
#22863=CARTESIAN_POINT ( 'NONE',  ( -8.049105076161786076E-16, 35.79101562608394005, -13.14518615778179544 ) ) ;
#22869=CARTESIAN_POINT ( 'NONE',  ( 13.57481594606304753, 34.30273437500000000, -5.622872871577873077 ) ) ;
#22870=CARTESIAN_POINT ( 'NONE',  ( 5.444914386472302859, 33.65781250108393152, 13.14518615778179189 ) ) ;
#22884=CARTESIAN_POINT ( 'NONE',  ( -8.312177448680279460E-16, 34.45156249999999432, -13.57481594606304576 ) ) ;
#22893=CARTESIAN_POINT ( 'NONE',  ( -8.312177448680279460E-16, 40.80156249999999574, -13.57481594606304576 ) ) ;
#22894=EDGE_CURVE ( 'NONE', #2116, #24154, #8718, .T. ) ;
#22903=CARTESIAN_POINT ( 'NONE',  ( 13.14518615778179900, 32.46718750108393436, -5.444914386472297529 ) ) ;
#22904=CARTESIAN_POINT ( 'NONE',  ( -13.57481594606304576, 35.59257812716788294, 5.622872871577880183 ) ) ;
#22929=CARTESIAN_POINT ( 'NONE',  ( 13.14518615778179900, 33.06250000108393294, -5.444914386472297529 ) ) ;
#22932=FACE_OUTER_BOUND ( 'NONE', #2006, .T. ) ;
#22949=AXIS2_PLACEMENT_3D ( 'NONE', #371, #18023, #15454 ) ;
#22954=EDGE_CURVE ( 'NONE', #8402, #25384, #20391, .T. ) ;
#22963=CARTESIAN_POINT ( 'NONE',  ( 6.944423533878893551, 31.68536041724614449, -11.16113349551710066 ) ) ;
#22973=CARTESIAN_POINT ( 'NONE',  ( 5.622872871577742515, 39.66054687500000142, 13.57481594606318076 ) ) ;
#22979=CARTESIAN_POINT ( 'NONE',  ( 1.907364849565526780E-15, 40.99999999999999289, 15.57481594606304576 ) ) ;
#22987=CARTESIAN_POINT ( 'NONE',  ( 5.444914386472297529, 40.30546875108393579, -13.14518615778179722 ) ) ;
#22993=CARTESIAN_POINT ( 'NONE',  ( -5.444914386472299306, 32.16953125108393152, 13.14518615778179722 ) ) ;
#23000=CARTESIAN_POINT ( 'NONE',  ( 13.14518615778179722, 34.05468750108394005, -5.444914386472297529 ) ) ;
#23007=CARTESIAN_POINT ( 'NONE',  ( 13.14518615778179900, 32.26875000108393721, -5.444914386472297529 ) ) ;
#23011=CARTESIAN_POINT ( 'NONE',  ( 9.598844408820456309, 35.14609374999999858, -9.598844408820458085 ) ) ;
#23023=ADVANCED_FACE ( 'NONE', ( #406 ), #16057, .F. ) ;
#23041=CARTESIAN_POINT ( 'NONE',  ( -8.312177448680279460E-16, 38.42031249999999432, -13.57481594606304576 ) ) ;
#23042=CARTESIAN_POINT ( 'NONE',  ( -8.049105076161786076E-16, 38.76757812608393294, -13.14518615778179544 ) ) ;
#23059=CARTESIAN_POINT ( 'NONE',  ( -5.622872871577828668, 32.51679687716787015, 13.57481594606309194 ) ) ;
#23061=CARTESIAN_POINT ( 'NONE',  ( 9.598844408820459861, 40.50390624999999289, 9.598844408820456309 ) ) ;
#23065=DIRECTION ( 'NONE',  ( 0.000000000000000000, 0.000000000000000000, -1.000000000000000000 ) ) ;
#23077=ORIENTED_EDGE ( 'NONE', *, *, #3949, .F. ) ;
#23079=CARTESIAN_POINT ( 'NONE',  ( -8.049105076161786076E-16, 40.55351562608393579, -13.14518615778179544 ) ) ;
#23080=CARTESIAN_POINT ( 'NONE',  ( -13.57481594606304576, 40.30546875216787583, 0.000000000000000000 ) ) ;
#23117=ADVANCED_FACE ( 'NONE', ( #6942 ), #22350, .F. ) ;
#23125=CARTESIAN_POINT ( 'NONE',  ( -13.14518615778179189, 38.22187500108393721, 5.444914386472304635 ) ) ;
#23132=CARTESIAN_POINT ( 'NONE',  ( 13.14518615778179900, 33.95546875108393436, 5.444914386472293977 ) ) ;
#23137=CARTESIAN_POINT ( 'NONE',  ( 5.622872871577786924, 32.51679687499999716, 13.57481594606313813 ) ) ;
#23146=CARTESIAN_POINT ( 'NONE',  ( -9.598844408820458085, 32.16953124999999147, -9.598844408820458085 ) ) ;
#23147=CARTESIAN_POINT ( 'NONE',  ( -13.14518615778179189, 31.87187500108393223, 5.444914386472304635 ) ) ;
#23167=CARTESIAN_POINT ( 'NONE',  ( 0.000000000000000000, 40.99999999999999289, 0.000000000000000000 ) ) ;
#23180=CARTESIAN_POINT ( 'NONE',  ( -13.57481594606304753, 39.36289062499999858, -5.622872871577873077 ) ) ;
#23181=CARTESIAN_POINT ( 'NONE',  ( -13.14518615778179900, 39.71015625108393010, -5.444914386472297529 ) ) ;
#23190=DIRECTION ( 'NONE',  ( -0.000000000000000000, -1.000000000000000000, -0.000000000000000000 ) ) ;
#23218=CARTESIAN_POINT ( 'NONE',  ( -13.14518615778179189, 40.00781250108393294, 5.444914386472304635 ) ) ;
#23219=CARTESIAN_POINT ( 'NONE',  ( 5.622872871577878406, 38.96601562716787015, 13.57481594606304576 ) ) ;
#23254=ORIENTED_EDGE ( 'NONE', *, *, #10156, .T. ) ;
#23263=CARTESIAN_POINT ( 'NONE',  ( -5.444914386472299306, 38.32109375108394289, 13.14518615778179722 ) ) ;
#23310=CARTESIAN_POINT ( 'NONE',  ( 0.000000000000000000, 40.99999999999999289, 0.000000000000000000 ) ) ;
#23316=CARTESIAN_POINT ( 'NONE',  ( 9.598844408820459861, 40.50390624999999289, 9.598844408820456309 ) ) ;
#23317=CARTESIAN_POINT ( 'NONE',  ( -13.57481594606304576, 31.62382812716787228, 5.622872871577880183 ) ) ;
#23321=EDGE_CURVE ( 'NONE', #2000, #11798, #13265, .T. ) ;
#23348=CARTESIAN_POINT ( 'NONE',  ( -8.312177448680279460E-16, 40.80156249999999574, -13.57481594606304576 ) ) ;
#23353=CARTESIAN_POINT ( 'NONE',  ( -9.295050272127044266, 39.26367187608393294, 9.295050272127047819 ) ) ;
#23371=CARTESIAN_POINT ( 'NONE',  ( -8.049105076161786076E-16, 39.56132812608393579, -13.14518615778179544 ) ) ;
#23384=ORIENTED_EDGE ( 'NONE', *, *, #18989, .T. ) ;
#23391=CARTESIAN_POINT ( 'NONE',  ( 2.493653234604083739E-15, 33.36015625216786873, 13.57481594606304576 ) ) ;
#23397=CARTESIAN_POINT ( 'NONE',  ( 9.295050272127046043, 38.66835937608393436, -9.295050272127046043 ) ) ;
#23407=CARTESIAN_POINT ( 'NONE',  ( -5.444914386472299306, 32.96328125108393436, 13.14518615778179722 ) ) ;
#23421=CARTESIAN_POINT ( 'NONE',  ( -5.622872871577873966, 32.11992187499999574, -13.57481594606304753 ) ) ;
#23422=EDGE_LOOP ( 'NONE', ( #13824, #14831, #10288, #4846 ) ) ;
#23438=CARTESIAN_POINT ( 'NONE',  ( 13.14518615778179900, 34.55078125108393294, 5.444914386472293977 ) ) ;
#23441=CARTESIAN_POINT ( 'NONE',  ( -8.312177448680279460E-16, 40.00781250000000000, -13.57481594606304576 ) ) ;
#23452=CARTESIAN_POINT ( 'NONE',  ( 5.622872871577871301, 39.95820312499999716, -13.57481594606304753 ) ) ;
#23453=CARTESIAN_POINT ( 'NONE',  ( -9.295050272127046043, 38.86679687608393863, -9.295050272127046043 ) ) ;
#23471=CARTESIAN_POINT ( 'NONE',  ( -13.57481594606304753, 36.98164062499999005, -5.622872871577872189 ) ) ;
#23490=CARTESIAN_POINT ( 'NONE',  ( -8.049105076161786076E-16, 38.96601562608393721, -13.14518615778179544 ) ) ;
#23504=( BOUNDED_CURVE ( )  B_SPLINE_CURVE ( 2, ( #6123, #23652, #18947, #18814, #4127, #12507, #20824, #19229, #27521 ),
 .UNSPECIFIED., .F., .F. ) 
 B_SPLINE_CURVE_WITH_KNOTS ( ( 3, 2, 2, 2, 3 ),
 ( 0.5208333333333332593, 0.5312500000000000000, 0.5416666666666667407, 0.5520833333333337034, 0.5625000000000004441 ),
 .UNSPECIFIED. ) 
 CURVE ( )  GEOMETRIC_REPRESENTATION_ITEM ( )  RATIONAL_B_SPLINE_CURVE ( ( 1.000000000000000888, 0.9238795325112859613, 1.000000000000000000, 0.9238795325112867385, 1.000000000000000000, 0.9238795325112867385, 1.000000000000000000, 0.9238795325112835188, 1.000000000000003331 ) ) 
 REPRESENTATION_ITEM ( '' )  );
#23509=CARTESIAN_POINT ( 'NONE',  ( -13.14518615778179900, 40.50390625108394005, -5.444914386472297529 ) ) ;
#23528=VERTEX_POINT ( 'NONE', #28024 ) ;
#23537=CARTESIAN_POINT ( 'NONE',  ( -13.14518615778179722, 38.91640625108393436, -5.444914386472297529 ) ) ;
#23562=EDGE_LOOP ( 'NONE', ( #12022, #27234, #21246, #19213 ) ) ;
#23564=PLANE ( 'NONE',  #17341 ) ;
#23577=CARTESIAN_POINT ( 'NONE',  ( 5.444914386472302859, 34.45156250108393436, 13.14518615778179189 ) ) ;
#23585=CIRCLE ( 'NONE', #13094, 13.57481594606304576 ) ;
#23587=EDGE_CURVE ( 'NONE', #21530, #10042, #25212, .T. ) ;
#23588=CARTESIAN_POINT ( 'NONE',  ( -8.312177448680279460E-16, 40.00781250000000000, -13.57481594606304576 ) ) ;
#23589=CARTESIAN_POINT ( 'NONE',  ( 13.14518615778179544, 40.15664062608393436, -1.609821015232357215E-15 ) ) ;
#23608=DIRECTION ( 'NONE',  ( 1.000000000000000000, 0.000000000000000000, 0.000000000000000000 ) ) ;
#23630=CARTESIAN_POINT ( 'NONE',  ( -13.14518615778179544, 40.75195312608393294, 0.000000000000000000 ) ) ;
#23642=CARTESIAN_POINT ( 'NONE',  ( -5.622872871577839327, 38.76757812499998579, 13.57481594606308128 ) ) ;
#23650=CARTESIAN_POINT ( 'NONE',  ( 9.295050272127046043, 38.66835937608393436, -9.295050272127046043 ) ) ;
#23652=CARTESIAN_POINT ( 'NONE',  ( 5.622872871577825116, 35.98945312500000426, -13.57481594606309372 ) ) ;
#23677=CARTESIAN_POINT ( 'NONE',  ( 13.14518615778179722, 36.23750000108393010, -5.444914386472297529 ) ) ;
#23691=DIRECTION ( 'NONE',  ( 0.000000000000000000, 0.000000000000000000, -1.000000000000000000 ) ) ;
#23696=CARTESIAN_POINT ( 'NONE',  ( -13.14518615778179189, 32.07031250108393294, 5.444914386472304635 ) ) ;
#23712=CARTESIAN_POINT ( 'NONE',  ( 5.622872871577946796, 37.27929687499999289, 13.57481594606297115 ) ) ;
#23718=CARTESIAN_POINT ( 'NONE',  ( -13.14518615778179544, 39.95820312608393010, 0.000000000000000000 ) ) ;
#23727=CARTESIAN_POINT ( 'NONE',  ( -9.598844408820458085, 37.72578124999999005, -9.598844408820458085 ) ) ;
#23731=CARTESIAN_POINT ( 'NONE',  ( 9.598844408820456309, 36.73359374999999716, -9.598844408820458085 ) ) ;
#23732=CARTESIAN_POINT ( 'NONE',  ( 13.14518615778179544, 36.18789062608393436, -1.609821015232357215E-15 ) ) ;
#23751=DIRECTION ( 'NONE',  ( -0.000000000000000000, -1.000000000000000000, -0.000000000000000000 ) ) ;
#23766=CARTESIAN_POINT ( 'NONE',  ( -5.444914386472299306, 36.93203125108394147, 13.14518615778179722 ) ) ;
#23767=CARTESIAN_POINT ( 'NONE',  ( -5.622872871577873077, 38.07304687716787583, 13.57481594606304753 ) ) ;
#23784=CARTESIAN_POINT ( 'NONE',  ( -13.14518615778179544, 38.17226562608393436, 0.000000000000000000 ) ) ;
#23793=CARTESIAN_POINT ( 'NONE',  ( -8.312177448680279460E-16, 40.00781250000000000, -13.57481594606304576 ) ) ;
#23810=UNCERTAINTY_MEASURE_WITH_UNIT (LENGTH_MEASURE( 1.000000000000000082E-05 ), #15640, 'distance_accuracy_value', 'NONE');
#23812=CARTESIAN_POINT ( 'NONE',  ( -5.444914386472297529, 35.64218750108393152, -13.14518615778179722 ) ) ;
#23816=ORIENTED_EDGE ( 'NONE', *, *, #3756, .T. ) ;
#23845=CARTESIAN_POINT ( 'NONE',  ( 5.622872871577786924, 33.40976562716787157, 13.57481594606313813 ) ) ;
#23854=CARTESIAN_POINT ( 'NONE',  ( 5.444914386472297529, 40.50390625108394005, -13.14518615778179900 ) ) ;
#23860=CARTESIAN_POINT ( 'NONE',  ( 13.14518615778179722, 37.92421875108393436, 5.444914386472293977 ) ) ;
#23862=CARTESIAN_POINT ( 'NONE',  ( -13.57481594606304398, 37.87460937499999147, 5.622872871577880183 ) ) ;
#23867=CARTESIAN_POINT ( 'NONE',  ( -9.598844408820454532, 35.54296874999999289, 9.598844408820459861 ) ) ;
#23868=CARTESIAN_POINT ( 'NONE',  ( -13.14518615778179189, 38.22187500108393010, 5.444914386472304635 ) ) ;
#23877=DIRECTION ( 'NONE',  ( 0.000000000000000000, 0.000000000000000000, -1.000000000000000000 ) ) ;
#23886=CARTESIAN_POINT ( 'NONE',  ( 2.493653234604083739E-15, 37.22968749999999716, 13.57481594606304576 ) ) ;
#23904=CARTESIAN_POINT ( 'NONE',  ( -13.14518615778179900, 36.73359375108393010, -5.444914386472297529 ) ) ;
#23905=CARTESIAN_POINT ( 'NONE',  ( -13.57481594606304753, 38.66835937716786731, -5.622872871577873077 ) ) ;
#23908=VECTOR ( 'NONE', #24773, 1000.000000000000000 ) ;
#23921=LINE ( 'NONE', #17359, #891 ) ;
#23926=CARTESIAN_POINT ( 'NONE',  ( -13.14518615778179189, 39.01562500108393294, 5.444914386472304635 ) ) ;
#23929=CARTESIAN_POINT ( 'NONE',  ( 5.622872871577928144, 39.16445312500000142, -13.57481594606299247 ) ) ;
#23949=ORIENTED_EDGE ( 'NONE', *, *, #10285, .F. ) ;
#23955=CARTESIAN_POINT ( 'NONE',  ( -13.14518615778179189, 35.04687500108393294, 5.444914386472304635 ) ) ;
#23982=DIRECTION ( 'NONE',  ( 0.000000000000000000, -0.000000000000000000, 1.000000000000000000 ) ) ;
#24000=CARTESIAN_POINT ( 'NONE',  ( 2.414731522848535132E-15, 37.77539062608393294, 13.14518615778179544 ) ) ;
#24005=CARTESIAN_POINT ( 'NONE',  ( 13.14518615778179722, 37.13046875108393863, 5.444914386472293977 ) ) ;
#24011=CARTESIAN_POINT ( 'NONE',  ( 2.493653234604083739E-15, 38.02343749999999289, 13.57481594606304576 ) ) ;
#24012=CARTESIAN_POINT ( 'NONE',  ( -5.444914386472297529, 38.02343750108394005, -13.14518615778179900 ) ) ;
#24028=DIRECTION ( 'NONE',  ( 0.000000000000000000, 0.000000000000000000, 1.000000000000000000 ) ) ;
#24048=CARTESIAN_POINT ( 'NONE',  ( -5.444914386472297529, 36.63437500108393152, -13.14518615778179900 ) ) ;
#24049=CARTESIAN_POINT ( 'NONE',  ( -13.57481594606304753, 37.08085937716786873, -5.622872871577873077 ) ) ;
#24067=CARTESIAN_POINT ( 'NONE',  ( -13.14518615778179900, 35.74140625108393721, -5.444914386472297529 ) ) ;
#24070=CARTESIAN_POINT ( 'NONE',  ( 5.622872871577912157, 38.86679687500001279, 13.57481594606301023 ) ) ;
#24095=CARTESIAN_POINT ( 'NONE',  ( -8.049105076161786076E-16, 34.79882812608393294, -13.14518615778179544 ) ) ;
#24096=CARTESIAN_POINT ( 'NONE',  ( 5.622872871577870413, 36.88242187716787157, -13.57481594606304753 ) ) ;
#24137=CARTESIAN_POINT ( 'NONE',  ( -9.295050272127044266, 39.26367187608393294, 9.295050272127047819 ) ) ;
#24145=CARTESIAN_POINT ( 'NONE',  ( 9.295050272127047819, 39.46210937608393721, 9.295050272127046043 ) ) ;
#24152=CARTESIAN_POINT ( 'NONE',  ( -13.57481594606304576, 37.82499999999999574, 0.000000000000000000 ) ) ;
#24153=CARTESIAN_POINT ( 'NONE',  ( -8.049105076161786076E-16, 37.97382812608393721, -13.14518615778179544 ) ) ;
#24154=VERTEX_POINT ( 'NONE', #27925 ) ;
#24165=FACE_BOUND ( 'NONE', #15831, .T. ) ;
#24189=CARTESIAN_POINT ( 'NONE',  ( 5.444914386472302859, 37.82500000108392868, 13.14518615778179189 ) ) ;
#24190=CARTESIAN_POINT ( 'NONE',  ( 9.598844408820459861, 37.42812500216787441, 9.598844408820456309 ) ) ;
#24194=ORIENTED_EDGE ( 'NONE', *, *, #3949, .T. ) ;
#24210=CARTESIAN_POINT ( 'NONE',  ( 5.444914386472297529, 37.13046875108393152, -13.14518615778179900 ) ) ;
#24235=CARTESIAN_POINT ( 'NONE',  ( -5.444914386472299306, 35.93984375108392726, 13.14518615778179722 ) ) ;
#24251=AXIS2_PLACEMENT_3D ( 'NONE', #21799, #22081, #2278 ) ;
#24262=DIRECTION ( 'NONE',  ( 0.000000000000000000, 0.000000000000000000, -1.000000000000000000 ) ) ;
#24278=CARTESIAN_POINT ( 'NONE',  ( -9.295050272127046043, 37.47773437608393010, -9.295050272127046043 ) ) ;
#24283=CARTESIAN_POINT ( 'NONE',  ( -5.444914386472297529, 37.42812500108394147, -13.14518615778179722 ) ) ;
#24290=CARTESIAN_POINT ( 'NONE',  ( 5.622872871577871301, 35.19570312499999432, -13.57481594606304753 ) ) ;
#24291=CARTESIAN_POINT ( 'NONE',  ( 5.444914386472302859, 37.62656250108393863, 13.14518615778179189 ) ) ;
#24326=CARTESIAN_POINT ( 'NONE',  ( -5.444914386472299306, 36.13828125108393863, 13.14518615778179722 ) ) ;
#24327=CARTESIAN_POINT ( 'NONE',  ( 9.598844408820456309, 37.62656250216787157, -9.598844408820458085 ) ) ;
#24345=CARTESIAN_POINT ( 'NONE',  ( -9.295050272127046043, 36.48554687608393721, -9.295050272127046043 ) ) ;
#24349=FACE_OUTER_BOUND ( 'NONE', #14753, .T. ) ;
#24367=ORIENTED_EDGE ( 'NONE', *, *, #26815, .T. ) ;
#24374=CARTESIAN_POINT ( 'NONE',  ( 13.14518615778179722, 34.55078125108393294, 5.444914386472293977 ) ) ;
#24416=CARTESIAN_POINT ( 'NONE',  ( -5.444914386472299306, 34.55078125108393294, 13.14518615778179722 ) ) ;
#24423=CARTESIAN_POINT ( 'NONE',  ( 13.14518615778179544, 38.76757812608393294, -1.609821015232357215E-15 ) ) ;
#24430=CARTESIAN_POINT ( 'NONE',  ( -9.598844408820458085, 34.55078124999999289, -9.598844408820458085 ) ) ;
#24431=CARTESIAN_POINT ( 'NONE',  ( -9.295050272127044266, 34.30273437608393294, 9.295050272127047819 ) ) ;
#24445=CARTESIAN_POINT ( 'NONE',  ( 13.57481594606304576, 36.63437499999999858, -1.662435489736055892E-15 ) ) ;
#24470=CARTESIAN_POINT ( 'NONE',  ( 9.295050272127047819, 32.31835937608393294, 9.295050272127046043 ) ) ;
#24471=CARTESIAN_POINT ( 'NONE',  ( 13.57481594606304576, 34.35234375216787583, -1.662435489736055892E-15 ) ) ;
#24491=CARTESIAN_POINT ( 'NONE',  ( 2.414731522848535132E-15, 37.57695312608392868, 13.14518615778179544 ) ) ;
#24495=CARTESIAN_POINT ( 'NONE',  ( -13.57481594606304398, 35.49335937499999005, 5.622872871577880183 ) ) ;
#24520=ORIENTED_EDGE ( 'NONE', *, *, #27964, .T. ) ;
#24521=CARTESIAN_POINT ( 'NONE',  ( 13.14518615778179722, 33.75703125108393010, 5.444914386472293977 ) ) ;
#24564=CARTESIAN_POINT ( 'NONE',  ( -8.049105076161786076E-16, 36.58476562608393579, -13.14518615778179544 ) ) ;
#24569=CARTESIAN_POINT ( 'NONE',  ( 5.444914386472297529, 33.36015625108393579, -13.14518615778179722 ) ) ;
#24576=CARTESIAN_POINT ( 'NONE',  ( 2.493653234604083739E-15, 34.84843749999999574, 13.57481594606304576 ) ) ;
#24577=CARTESIAN_POINT ( 'NONE',  ( 13.14518615778179900, 32.96328125108393436, 5.444914386472293977 ) ) ;
#24609=CARTESIAN_POINT ( 'NONE',  ( 13.57481594606304576, 35.14609375216787157, -1.662435489736055892E-15 ) ) ;
#24615=CARTESIAN_POINT ( 'NONE',  ( 5.444914386472297529, 33.36015625108393579, -13.14518615778179900 ) ) ;
#24616=CARTESIAN_POINT ( 'NONE',  ( -13.57481594606304753, 33.90585937716787868, -5.622872871577873077 ) ) ;
#24637=CARTESIAN_POINT ( 'NONE',  ( -5.444914386472297529, 37.22968750108393721, -13.14518615778179900 ) ) ;
#24642=CARTESIAN_POINT ( 'NONE',  ( -5.622872871577964560, 37.77539062716787299, -13.57481594606295339 ) ) ;
#24643=CARTESIAN_POINT ( 'NONE',  ( -13.57481594606304753, 35.39414062499999147, -5.622872871577872189 ) ) ;
#24666=CARTESIAN_POINT ( 'NONE',  ( 9.295050272127047819, 33.70742187608393436, 9.295050272127046043 ) ) ;
#24667=CARTESIAN_POINT ( 'NONE',  ( -8.312177448680279460E-16, 32.07031249999999289, -13.57481594606304576 ) ) ;
#24706=CARTESIAN_POINT ( 'NONE',  ( 13.14518615778179900, 34.74921875108395142, 5.444914386472293977 ) ) ;
#24714=CARTESIAN_POINT ( 'NONE',  ( -5.444914386472297529, 33.45937500108394147, -13.14518615778179722 ) ) ;
#24716=CARTESIAN_POINT ( 'NONE',  ( -13.57481594606304398, 36.28710937499999289, 5.622872871577880183 ) ) ;
#24720=CARTESIAN_POINT ( 'NONE',  ( -5.622872871577873077, 32.41757812499999858, 13.57481594606304753 ) ) ;
#24721=CARTESIAN_POINT ( 'NONE',  ( 2.414731522848535132E-15, 32.81445312608393294, 13.14518615778179544 ) ) ;
#24733=CARTESIAN_POINT ( 'NONE',  ( 13.57481594606304931, 36.58476562499999574, 5.622872871577868636 ) ) ;
#24747=CARTESIAN_POINT ( 'NONE',  ( 13.57481594606304931, 35.09648437716787583, 5.622872871577868636 ) ) ;
#24752=CARTESIAN_POINT ( 'NONE',  ( 13.14518615778179544, 33.21132812608393436, -1.609821015232357215E-15 ) ) ;
#24753=CARTESIAN_POINT ( 'NONE',  ( 5.622872871577871301, 33.70742187716787441, -13.57481594606304753 ) ) ;
#24773=DIRECTION ( 'NONE',  ( -0.000000000000000000, -1.000000000000000000, -0.000000000000000000 ) ) ;
#24775=CARTESIAN_POINT ( 'NONE',  ( -9.295050272127044266, 34.30273437608393294, 9.295050272127047819 ) ) ;
#24778=CARTESIAN_POINT ( 'NONE',  ( -9.598844408820458085, 37.82500000216787583, -9.598844408820458085 ) ) ;
#24795=VERTEX_POINT ( 'NONE', #6532 ) ;
#24799=EDGE_CURVE ( 'NONE', #19746, #2116, #17284, .T. ) ;
#24803=CARTESIAN_POINT ( 'NONE',  ( -13.14518615778179189, 34.25312500108393721, 5.444914386472304635 ) ) ;
#24822=ADVANCED_FACE ( 'NONE', ( #24349 ), #8816, .F. ) ;
#24837=EDGE_CURVE ( 'NONE', #6267, #3669, #15109, .T. ) ;
#24849=CARTESIAN_POINT ( 'NONE',  ( 5.444914386472297529, 34.94765625108394147, -13.14518615778179900 ) ) ;
#24854=CARTESIAN_POINT ( 'NONE',  ( -13.14518615778179722, 34.35234375108393579, -5.444914386472297529 ) ) ;
#24859=CARTESIAN_POINT ( 'NONE',  ( 5.622872871577878406, 34.89804687499999147, 13.57481594606304576 ) ) ;
#24860=CARTESIAN_POINT ( 'NONE',  ( 5.444914386472297529, 35.54296875108393294, -13.14518615778179900 ) ) ;
#24879=ORIENTED_EDGE ( 'NONE', *, *, #470, .F. ) ;
#24896=CARTESIAN_POINT ( 'NONE',  ( -9.295050272127044266, 33.70742187608393436, 9.295050272127047819 ) ) ;
#24897=CARTESIAN_POINT ( 'NONE',  ( -5.622872871577873077, 34.10429687716786873, 13.57481594606304753 ) ) ;
#24902=CARTESIAN_POINT ( 'NONE',  ( -8.312177448680279460E-16, 32.07031249999999289, -13.57481594606304576 ) ) ;
#24916=CARTESIAN_POINT ( 'NONE',  ( -9.295050272127044266, 31.92148437608393508, 9.295050272127047819 ) ) ;
#24919=CARTESIAN_POINT ( 'NONE',  ( 9.598844408820459861, 37.42812500216787441, 9.598844408820456309 ) ) ;
#24920=CARTESIAN_POINT ( 'NONE',  ( -5.622872871578057818, 35.59257812499998863, 13.57481594606286457 ) ) ;
#24938=VECTOR ( 'NONE', #4642, 1000.000000000000000 ) ;
#24943=CARTESIAN_POINT ( 'NONE',  ( 9.295050272127047819, 34.50117187608393010, 9.295050272127046043 ) ) ;
#24958=CARTESIAN_POINT ( 'NONE',  ( 9.598844408820456309, 39.90859374999999432, -9.598844408820458085 ) ) ;
#24985=CARTESIAN_POINT ( 'NONE',  ( 13.57481594606304753, 38.37070312716787157, -5.622872871577873966 ) ) ;
#24986=CARTESIAN_POINT ( 'NONE',  ( -9.295050272127046043, 32.71523437608393436, -9.295050272127046043 ) ) ;
#24988=EDGE_CURVE ( 'NONE', #21956, #34, #8550, .T. ) ;
#24995=CARTESIAN_POINT ( 'NONE',  ( -9.295050272127044266, 36.08867187608393579, 9.295050272127047819 ) ) ;
#25000=CARTESIAN_POINT ( 'NONE',  ( 13.57481594606304931, 32.61601562499999574, 5.622872871577869525 ) ) ;
#25001=CARTESIAN_POINT ( 'NONE',  ( 5.444914386472302859, 34.45156250108393436, 13.14518615778179189 ) ) ;
#25007=CARTESIAN_POINT ( 'NONE',  ( 9.598844408820456309, 32.86406250216787583, -9.598844408820458085 ) ) ;
#25028=DIRECTION ( 'NONE',  ( 0.000000000000000000, 0.000000000000000000, 1.000000000000000000 ) ) ;
#25036=CARTESIAN_POINT ( 'NONE',  ( 5.444914386472302859, 32.26875000108393721, 13.14518615778179189 ) ) ;
#25037=CARTESIAN_POINT ( 'NONE',  ( -9.598844408820458085, 35.44375000216787441, -9.598844408820458085 ) ) ;
#25059=CARTESIAN_POINT ( 'NONE',  ( 9.295050272127047819, 34.50117187608393010, 9.295050272127046043 ) ) ;
#25064=CARTESIAN_POINT ( 'NONE',  ( -9.598844408820454532, 35.54296874999999289, 9.598844408820459861 ) ) ;
#25082=ORIENTED_EDGE ( 'NONE', *, *, #6344, .F. ) ;
#25095=CARTESIAN_POINT ( 'NONE',  ( 13.57481594606304931, 35.89023437716787868, 5.622872871577868636 ) ) ;
#25115=CARTESIAN_POINT ( 'NONE',  ( 5.444914386472297529, 37.92421875108393436, -13.14518615778179722 ) ) ;
#25121=CARTESIAN_POINT ( 'NONE',  ( 2.414731522848535132E-15, 33.01289062608393721, 13.14518615778179544 ) ) ;
#25129=CARTESIAN_POINT ( 'NONE',  ( -9.295050272127046043, 34.30273437608393294, -9.295050272127046043 ) ) ;
#25134=CARTESIAN_POINT ( 'NONE',  ( 2.414731522848535132E-15, 32.02070312608393010, 13.14518615778179544 ) ) ;
#25150=ORIENTED_EDGE ( 'NONE', *, *, #23587, .F. ) ;
#25167=CARTESIAN_POINT ( 'NONE',  ( 9.598844408820456309, 40.70234374999999716, -9.598844408820458085 ) ) ;
#25168=CARTESIAN_POINT ( 'NONE',  ( -13.14518615778179900, 38.91640625108393436, -5.444914386472297529 ) ) ;
#25181=LINE ( 'NONE', #5669, #2681 ) ;
#25194=CARTESIAN_POINT ( 'NONE',  ( 13.14518615778179900, 33.85625000108393579, -5.444914386472297529 ) ) ;
#25212=CIRCLE ( 'NONE', #22949, 13.57481594606304576 ) ;
#25220=CARTESIAN_POINT ( 'NONE',  ( 7.171390501253594785, 31.30502191632583830, -11.52591802191987114 ) ) ;
#25240=AXIS2_PLACEMENT_3D ( 'NONE', #17840, #20127, #7424 ) ;
#25251=CARTESIAN_POINT ( 'NONE',  ( 5.444914386472302859, 38.42031250108393436, 13.14518615778179189 ) ) ;
#25256=CARTESIAN_POINT ( 'NONE',  ( 0.000000000000000000, 30.99999999999999645, 0.000000000000000000 ) ) ;
#25258=CARTESIAN_POINT ( 'NONE',  ( -13.14518615778179900, 33.55859375108393294, -5.444914386472297529 ) ) ;
#25262=CARTESIAN_POINT ( 'NONE',  ( 13.57481594606304576, 32.66562499999999858, -1.662435489736055892E-15 ) ) ;
#25265=CARTESIAN_POINT ( 'NONE',  ( 2.414731522848535132E-15, 33.01289062608393721, 13.14518615778179544 ) ) ;
#25273=CARTESIAN_POINT ( 'NONE',  ( -5.444914386472297529, 31.67343750108393863, -13.14518615778179900 ) ) ;
#25307=CARTESIAN_POINT ( 'NONE',  ( 13.57481594606304576, 39.80937499999999574, -1.662435489736055892E-15 ) ) ;
#25308=CARTESIAN_POINT ( 'NONE',  ( 13.57481594606304931, 31.92148437716787512, 5.622872871577869525 ) ) ;
#25326=LINE ( 'NONE', #16768, #27746 ) ;
#25328=CARTESIAN_POINT ( 'NONE',  ( -9.598844408820458085, 32.26875000216787726, -9.598844408820458085 ) ) ;
#25343=CARTESIAN_POINT ( 'NONE',  ( -8.312177448680279460E-16, 33.65781249999999147, -13.57481594606304576 ) ) ;
#25349=CARTESIAN_POINT ( 'NONE',  ( 13.14518615778179900, 40.30546875108393579, 5.444914386472293977 ) ) ;
#25354=ADVANCED_FACE ( 'NONE', ( #19011, #8044 ), #7772, .T. ) ;
#25355=AXIS2_PLACEMENT_3D ( 'NONE', #9623, #18328, #11886 ) ;
#25384=VERTEX_POINT ( 'NONE', #25995 ) ;
#25398=CARTESIAN_POINT ( 'NONE',  ( 13.14518615778179722, 40.20625000108393010, -5.444914386472297529 ) ) ;
#25407=CARTESIAN_POINT ( 'NONE',  ( 9.295050272127047819, 33.90585937608393863, 9.295050272127046043 ) ) ;
#25430=CARTESIAN_POINT ( 'NONE',  ( -9.598844408820454532, 33.95546874999999432, 9.598844408820459861 ) ) ;
#25438=CARTESIAN_POINT ( 'NONE',  ( -13.57481594606304576, 40.20624999999999005, 0.000000000000000000 ) ) ;
#25442=CARTESIAN_POINT ( 'NONE',  ( 13.14518615778179544, 39.56132812608393579, -1.609821015232357215E-15 ) ) ;
#25450=CARTESIAN_POINT ( 'NONE',  ( -5.444914386472297529, 31.87187500108393223, -13.14518615778179900 ) ) ;
#25451=CARTESIAN_POINT ( 'NONE',  ( -9.598844408820458085, 32.26875000216787726, -9.598844408820458085 ) ) ;
#25483=CARTESIAN_POINT ( 'NONE',  ( -13.57481594606304576, 40.99999999999999289, 0.000000000000000000 ) ) ;
#25488=CARTESIAN_POINT ( 'NONE',  ( -13.14518615778179900, 39.90859375108394147, -5.444914386472297529 ) ) ;
#25489=CARTESIAN_POINT ( 'NONE',  ( 9.598844408820456309, 40.00781250216787299, -9.598844408820458085 ) ) ;
#25500=DIRECTION ( 'NONE',  ( -0.000000000000000000, -1.000000000000000000, -0.000000000000000000 ) ) ;
#25504=CARTESIAN_POINT ( 'NONE',  ( 6.944426393311537993, 31.75150625057403175, -11.16113171639042356 ) ) ;
#25507=CARTESIAN_POINT ( 'NONE',  ( 13.14518615778179900, 40.10703125108393152, 5.444914386472293977 ) ) ;
#25509=LINE ( 'NONE', #8118, #5530 ) ;
#25533=CARTESIAN_POINT ( 'NONE',  ( -9.295050272127046043, 40.45429687608393721, -9.295050272127046043 ) ) ;
#25544=CARTESIAN_POINT ( 'NONE',  ( 13.14518615778179544, 33.21132812608393436, -1.609821015232357215E-15 ) ) ;
#25552=CARTESIAN_POINT ( 'NONE',  ( -5.444914386472297529, 32.66562500108393863, -13.14518615778179722 ) ) ;
#25557=CARTESIAN_POINT ( 'NONE',  ( -8.312177448680279460E-16, 32.07031249999999289, -13.57481594606304576 ) ) ;
#25577=CARTESIAN_POINT ( 'NONE',  ( -9.295050272127044266, 40.05742187608393579, 9.295050272127047819 ) ) ;
#25583=CARTESIAN_POINT ( 'NONE',  ( 13.57481594606304576, 39.01562500000000000, -1.662435489736055892E-15 ) ) ;
#25584=CARTESIAN_POINT ( 'NONE',  ( -5.444914386472299306, 39.11484375108394573, 13.14518615778179722 ) ) ;
#25621=CARTESIAN_POINT ( 'NONE',  ( 9.295050272127047819, 38.66835937608393436, 9.295050272127046043 ) ) ;
#25622=CARTESIAN_POINT ( 'NONE',  ( -5.622872871577873077, 40.15664062716787441, -13.57481594606304753 ) ) ;
#25637=CARTESIAN_POINT ( 'NONE',  ( -5.444914386472299306, 38.32109375108394289, 13.14518615778179722 ) ) ;
#25653=ORIENTED_EDGE ( 'NONE', *, *, #16443, .F. ) ;
#25654=EDGE_CURVE ( 'NONE', #5311, #138, #13442, .T. ) ;
#25665=CARTESIAN_POINT ( 'NONE',  ( 13.14518615778179544, 39.36289062608393152, -1.609821015232357215E-15 ) ) ;
#25670=EDGE_LOOP ( 'NONE', ( #27665, #24520, #7862, #4250, #12254, #19537 ) ) ;
#25709=CARTESIAN_POINT ( 'NONE',  ( -5.444914386472297529, 33.26093750108393721, -13.14518615778179900 ) ) ;
#25719=EDGE_CURVE ( 'NONE', #1494, #2719, #4706, .T. ) ;
#25720=CARTESIAN_POINT ( 'NONE',  ( -13.57481594606304576, 39.41249999999999432, 0.000000000000000000 ) ) ;
#25721=CARTESIAN_POINT ( 'NONE',  ( -13.14518615778179544, 39.75976562608393294, 0.000000000000000000 ) ) ;
#25734=CARTESIAN_POINT ( 'NONE',  ( -13.57481594606304753, 34.60039062499999574, -5.622872871577872189 ) ) ;
#25757=ORIENTED_EDGE ( 'NONE', *, *, #11777, .T. ) ;
#25759=CARTESIAN_POINT ( 'NONE',  ( -13.14518615778179544, 39.16445312608393436, 0.000000000000000000 ) ) ;
#25760=CARTESIAN_POINT ( 'NONE',  ( -9.598844408820454532, 39.61093750216787868, 9.598844408820459861 ) ) ;
#25770=CARTESIAN_POINT ( 'NONE',  ( -5.622872871577964560, 38.46992187499999005, -13.57481594606295339 ) ) ;
#25778=CARTESIAN_POINT ( 'NONE',  ( 13.14518615778179900, 39.31328125108392868, 5.444914386472293977 ) ) ;
#25804=CARTESIAN_POINT ( 'NONE',  ( -13.14518615778179189, 35.84062500108394289, 5.444914386472304635 ) ) ;
#25826=CARTESIAN_POINT ( 'NONE',  ( 5.444914386472297529, 32.56640625108394005, -13.14518615778179722 ) ) ;
#25844=CARTESIAN_POINT ( 'NONE',  ( 9.598844408820459861, 37.32890624999999574, 9.598844408820456309 ) ) ;
#25850=CARTESIAN_POINT ( 'NONE',  ( 13.14518615778179900, 39.61093750108393863, -5.444914386472297529 ) ) ;
#25865=CARTESIAN_POINT ( 'NONE',  ( 9.598844408820459861, 38.12265624999999858, 9.598844408820456309 ) ) ;
#25866=CARTESIAN_POINT ( 'NONE',  ( 13.14518615778179544, 36.98164062608393010, -1.609821015232357215E-15 ) ) ;
#25878=EDGE_CURVE ( 'NONE', #3914, #18296, #26470, .T. ) ;
#25883=VECTOR ( 'NONE', #26175, 1000.000000000000000 ) ;
#25916=CARTESIAN_POINT ( 'NONE',  ( -13.57481594606304398, 38.66835937499999432, 5.622872871577880183 ) ) ;
#25923=CARTESIAN_POINT ( 'NONE',  ( -13.14518615778179189, 39.80937500108392868, 5.444914386472304635 ) ) ;
#25949=CARTESIAN_POINT ( 'NONE',  ( -5.444914386472297529, 36.43593750108394147, -13.14518615778179722 ) ) ;
#25987=DIRECTION ( 'NONE',  ( -0.000000000000000000, -1.000000000000000000, -0.000000000000000000 ) ) ;
#25992=CARTESIAN_POINT ( 'NONE',  ( -5.444914386472299306, 40.10703125108393152, 13.14518615778179722 ) ) ;
#25995=CARTESIAN_POINT ( 'NONE',  ( -8.312177448680279460E-16, 31.37578125216787583, -13.57481594606304576 ) ) ;
#25997=CARTESIAN_POINT ( 'NONE',  ( -5.444914386472297529, 39.01562500108394005, -13.14518615778179722 ) ) ;
#25999=CARTESIAN_POINT ( 'NONE',  ( -13.57481594606304576, 37.82499999999999574, 0.000000000000000000 ) ) ;
#26003=CARTESIAN_POINT ( 'NONE',  ( 13.57481594606304753, 35.89023437499999858, -5.622872871577873077 ) ) ;
#26004=CARTESIAN_POINT ( 'NONE',  ( 13.14518615778179544, 37.77539062608393294, -1.609821015232357215E-15 ) ) ;
#26013=CARTESIAN_POINT ( 'NONE',  ( 2.493653234604083739E-15, 38.91640625216786731, 13.57481594606304576 ) ) ;
#26040=CARTESIAN_POINT ( 'NONE',  ( -13.14518615778179900, 35.93984375108393436, -5.444914386472297529 ) ) ;
#26041=CARTESIAN_POINT ( 'NONE',  ( -13.57481594606304576, 37.13046875216787868, 0.000000000000000000 ) ) ;
#26043=EDGE_CURVE ( 'NONE', #25384, #6320, #9631, .T. ) ;
#26060=CARTESIAN_POINT ( 'NONE',  ( -13.14518615778179544, 40.55351562608393579, 0.000000000000000000 ) ) ;
#26081=CARTESIAN_POINT ( 'NONE',  ( -9.598844408820454532, 33.26093750216787726, 9.598844408820459861 ) ) ;
#26089=CARTESIAN_POINT ( 'NONE',  ( 2.414731522848535132E-15, 35.98945312608393010, 13.14518615778179544 ) ) ;
#26132=CARTESIAN_POINT ( 'NONE',  ( 9.295050272127046043, 40.45429687608393721, -9.295050272127046043 ) ) ;
#26137=CARTESIAN_POINT ( 'NONE',  ( -5.444914386472297529, 38.22187500108393721, -13.14518615778179722 ) ) ;
#26139=CARTESIAN_POINT ( 'NONE',  ( -8.312177448680279460E-16, 37.62656249999999858, -13.57481594606304576 ) ) ;
#26143=VECTOR ( 'NONE', #5483, 1000.000000000000000 ) ;
#26144=CARTESIAN_POINT ( 'NONE',  ( -8.312177448680279460E-16, 36.03906250000000000, -13.57481594606304576 ) ) ;
#26145=CARTESIAN_POINT ( 'NONE',  ( 9.295050272127047819, 37.67617187608393436, 9.295050272127046043 ) ) ;
#26169=CARTESIAN_POINT ( 'NONE',  ( -13.14518615778179544, 40.65273437608393436, 0.000000000000000000 ) ) ;
#26174=CARTESIAN_POINT ( 'NONE',  ( -5.622872871578011633, 39.56132812500000284, 13.57481594606290720 ) ) ;
#26175=DIRECTION ( 'NONE',  ( -0.000000000000000000, -1.000000000000000000, -0.000000000000000000 ) ) ;
#26180=CARTESIAN_POINT ( 'NONE',  ( -9.295050272127044266, 35.29492187608393294, 9.295050272127047819 ) ) ;
#26181=CARTESIAN_POINT ( 'NONE',  ( -8.312177448680279460E-16, 36.13828125216787157, -13.57481594606304576 ) ) ;
#26189=EDGE_CURVE ( 'NONE', #11798, #27263, #14207, .T. ) ;
#26193=FACE_OUTER_BOUND ( 'NONE', #2942, .T. ) ;
#26200=( BOUNDED_CURVE ( )  B_SPLINE_CURVE ( 2, ( #16184, #3226, #22187, #17903, #24609, #24747, #9629, #9769, #9350 ),
 .UNSPECIFIED., .F., .F. ) 
 B_SPLINE_CURVE_WITH_KNOTS ( ( 3, 2, 2, 2, 3 ),
 ( 0.5208333333333332593, 0.5312499999999997780, 0.5416666666666664076, 0.5520833333333330373, 0.5624999999999996669 ),
 .UNSPECIFIED. ) 
 CURVE ( )  GEOMETRIC_REPRESENTATION_ITEM ( )  RATIONAL_B_SPLINE_CURVE ( ( 1.000000000000000888, 0.9238795325112859613, 1.000000000000000000, 0.9238795325112867385, 1.000000000000000000, 0.9238795325112867385, 1.000000000000000000, 0.9238795325112891810, 0.9999999999999975575 ) ) 
 REPRESENTATION_ITEM ( '' )  );
#26202=CARTESIAN_POINT ( 'NONE',  ( -13.14518615778179544, 36.58476562608393579, 0.000000000000000000 ) ) ;
#26227=DIRECTION ( 'NONE',  ( -0.000000000000000000, -1.000000000000000000, -0.000000000000000000 ) ) ;
#26234=CARTESIAN_POINT ( 'NONE',  ( -9.295050272127046043, 34.89804687608393152, -9.295050272127046043 ) ) ;
#26254=ORIENTED_EDGE ( 'NONE', *, *, #22954, .F. ) ;
#26256=( BOUNDED_CURVE ( )  B_SPLINE_CURVE ( 2, ( #17580, #2209, #6746, #19583, #17440, #10872, #4623, #15431, #21876 ),
 .UNSPECIFIED., .F., .F. ) 
 B_SPLINE_CURVE_WITH_KNOTS ( ( 3, 2, 2, 2, 3 ),
 ( 0.06250000000000004163, 0.07291666666666665741, 0.08333333333333325932, 0.09374999999999987510, 0.1041666666666664909 ),
 .UNSPECIFIED. ) 
 CURVE ( )  GEOMETRIC_REPRESENTATION_ITEM ( )  RATIONAL_B_SPLINE_CURVE ( ( 0.9999999999999996669, 0.9238795325112870716, 1.000000000000000000, 0.9238795325112867385, 1.000000000000000000, 0.9238795325112867385, 1.000000000000000000, 0.9238795325112880708, 0.9999999999999986677 ) ) 
 REPRESENTATION_ITEM ( '' )  );
#26259=CARTESIAN_POINT ( 'NONE',  ( 0.000000000000000000, 40.99999999999999289, 0.000000000000000000 ) ) ;
#26276=VERTEX_POINT ( 'NONE', #7033 ) ;
#26277=ORIENTED_EDGE ( 'NONE', *, *, #4304, .T. ) ;
#26278=CARTESIAN_POINT ( 'NONE',  ( -8.049105076161786076E-16, 39.75976562608394005, -13.14518615778179544 ) ) ;
#26281=CARTESIAN_POINT ( 'NONE',  ( 9.598844408820459861, 38.12265624999999858, 9.598844408820456309 ) ) ;
#26285=CARTESIAN_POINT ( 'NONE',  ( 13.14518615778179722, 38.71796875108393721, 5.444914386472293977 ) ) ;
#26291=CARTESIAN_POINT ( 'NONE',  ( 9.598844408820456309, 37.52734375000000000, -9.598844408820458085 ) ) ;
#26292=CARTESIAN_POINT ( 'NONE',  ( -5.444914386472297529, 35.64218750108392442, -13.14518615778179900 ) ) ;
#26294=ORIENTED_EDGE ( 'NONE', *, *, #21282, .T. ) ;
#26309=( NAMED_UNIT ( * ) PLANE_ANGLE_UNIT ( ) SI_UNIT ( $, .RADIAN. ) );
#26315=VECTOR ( 'NONE', #2517, 1000.000000000000000 ) ;
#26329=CARTESIAN_POINT ( 'NONE',  ( 13.14518615778179544, 37.97382812608393721, -1.609821015232357215E-15 ) ) ;
#26330=CARTESIAN_POINT ( 'NONE',  ( 9.598844408820456309, 36.03906250216787299, -9.598844408820458085 ) ) ;
#26334=EDGE_CURVE ( 'NONE', #11263, #8015, #2247, .T. ) ;
#26351=CARTESIAN_POINT ( 'NONE',  ( -13.14518615778179544, 37.37851562608393863, 0.000000000000000000 ) ) ;
#26359=VERTEX_POINT ( 'NONE', #18017 ) ;
#26382=CARTESIAN_POINT ( 'NONE',  ( -5.444914386472299306, 37.52734375108393294, 13.14518615778179722 ) ) ;
#26383=CARTESIAN_POINT ( 'NONE',  ( 13.57481594606304931, 36.68398437716787441, 5.622872871577868636 ) ) ;
#26425=CARTESIAN_POINT ( 'NONE',  ( 5.444914386472297529, 38.91640625108393436, -13.14518615778179900 ) ) ;
#26430=CIRCLE ( 'NONE', #20061, 13.57481594606304576 ) ;
#26431=CARTESIAN_POINT ( 'NONE',  ( 9.295050272127046043, 38.07304687608393579, -9.295050272127046043 ) ) ;
#26436=CARTESIAN_POINT ( 'NONE',  ( 9.598844408820456309, 35.93984374999999432, -9.598844408820458085 ) ) ;
#26437=CARTESIAN_POINT ( 'NONE',  ( -8.049105076161786076E-16, 37.18007812608393436, -13.14518615778179544 ) ) ;
#26468=DIRECTION ( 'NONE',  ( -0.000000000000000000, -1.000000000000000000, -0.000000000000000000 ) ) ;
#26469=CARTESIAN_POINT ( 'NONE',  ( 0.000000000000000000, 40.99999999999999289, 0.000000000000000000 ) ) ;
#26470=LINE ( 'NONE', #242, #14232 ) ;
#26474=CARTESIAN_POINT ( 'NONE',  ( -9.598844408820458085, 40.20625000216787726, -9.598844408820458085 ) ) ;
#26475=CARTESIAN_POINT ( 'NONE',  ( 13.14518615778179900, 36.33671875108394289, 5.444914386472293977 ) ) ;
#26476=CARTESIAN_POINT ( 'NONE',  ( 13.57481594606304753, 36.78320312716786589, -5.622872871577873077 ) ) ;
#26495=CARTESIAN_POINT ( 'NONE',  ( -9.295050272127046043, 37.27929687608393294, -9.295050272127046043 ) ) ;
#26523=CARTESIAN_POINT ( 'NONE',  ( 5.444914386472302859, 32.86406250108392868, 13.14518615778179189 ) ) ;
#26524=CARTESIAN_POINT ( 'NONE',  ( -8.312177448680279460E-16, 36.93203125216787441, -13.57481594606304576 ) ) ;
#26566=CARTESIAN_POINT ( 'NONE',  ( -5.444914386472297529, 37.42812500108394147, -13.14518615778179900 ) ) ;
#26572=ADVANCED_FACE ( 'NONE', ( #17132 ), #10845, .F. ) ;
#26573=CARTESIAN_POINT ( 'NONE',  ( 5.444914386472297529, 36.53515625108394715, -13.14518615778179722 ) ) ;
#26574=EDGE_LOOP ( 'NONE', ( #21816, #22527, #12894, #14778 ) ) ;
#26578=ORIENTED_EDGE ( 'NONE', *, *, #11147, .T. ) ;
#26580=CARTESIAN_POINT ( 'NONE',  ( -9.598844408820458085, 33.75703124999999005, -9.598844408820458085 ) ) ;
#26581=CARTESIAN_POINT ( 'NONE',  ( -5.444914386472297529, 34.05468750108393294, -13.14518615778179900 ) ) ;
#26596=CARTESIAN_POINT ( 'NONE',  ( 9.598844408820456309, 36.73359374999999716, -9.598844408820458085 ) ) ;
#26621=CARTESIAN_POINT ( 'NONE',  ( -13.14518615778179900, 37.52734375108393294, -5.444914386472297529 ) ) ;
#26622=CARTESIAN_POINT ( 'NONE',  ( -5.622872871577873077, 38.56914062716788294, -13.57481594606304753 ) ) ;
#26641=CARTESIAN_POINT ( 'NONE',  ( -5.444914386472297529, 34.84843750108393579, -13.14518615778179900 ) ) ;
#26646=CARTESIAN_POINT ( 'NONE',  ( 2.493653234604083739E-15, 38.81718749999999574, 13.57481594606304576 ) ) ;
#26670=CARTESIAN_POINT ( 'NONE',  ( -8.049105076161786076E-16, 31.62382812608393579, -13.14518615778179544 ) ) ;
#26694=ADVANCED_FACE ( 'NONE', ( #14577 ), #27989, .T. ) ;
#26710=CARTESIAN_POINT ( 'NONE',  ( -13.14518615778179900, 35.14609375108393152, -5.444914386472297529 ) ) ;
#26717=CARTESIAN_POINT ( 'NONE',  ( -5.444914386472299306, 36.13828125108393152, 13.14518615778179722 ) ) ;
#26718=AXIS2_PLACEMENT_3D ( 'NONE', #16624, #23190, #7927 ) ;
#26722=AXIS2_PLACEMENT_3D ( 'NONE', #12964, #13102, #19549 ) ;
#26724=CARTESIAN_POINT ( 'NONE',  ( 9.598844408820456309, 34.35234374999999574, -9.598844408820458085 ) ) ;
#26725=CARTESIAN_POINT ( 'NONE',  ( 13.14518615778179544, 33.01289062608393010, -1.609821015232357215E-15 ) ) ;
#26757=CARTESIAN_POINT ( 'NONE',  ( 0.000000000000000000, 40.99999999999999289, -13.57481594606304576 ) ) ;
#26761=CARTESIAN_POINT ( 'NONE',  ( -9.295050272127046043, 35.09648437608393579, -9.295050272127046043 ) ) ;
#26762=CARTESIAN_POINT ( 'NONE',  ( 9.598844408820459861, 35.04687500216787299, 9.598844408820456309 ) ) ;
#26785=CARTESIAN_POINT ( 'NONE',  ( -9.295050272127044266, 36.68398437608392726, 9.295050272127047819 ) ) ;
#26805=ORIENTED_EDGE ( 'NONE', *, *, #23587, .T. ) ;
#26814=CARTESIAN_POINT ( 'NONE',  ( -13.14518615778179544, 32.61601562608393579, 0.000000000000000000 ) ) ;
#26815=EDGE_CURVE ( 'NONE', #17847, #3914, #16034, .T. ) ;
#26844=AXIS2_PLACEMENT_3D ( 'NONE', #8635, #24028, #23608 ) ;
#26851=( BOUNDED_CURVE ( )  B_SPLINE_CURVE ( 2, ( #21871, #19301, #11004, #17151, #21584, #28000, #26281, #17576, #21731 ),
 .UNSPECIFIED., .F., .F. ) 
 B_SPLINE_CURVE_WITH_KNOTS ( ( 3, 2, 2, 2, 3 ),
 ( 0.2708333333333330928, 0.2812499999999998890, 0.2916666666666666852, 0.3020833333333334259, 0.3125000000000002220 ),
 .UNSPECIFIED. ) 
 CURVE ( )  GEOMETRIC_REPRESENTATION_ITEM ( )  RATIONAL_B_SPLINE_CURVE ( ( 1.000000000000001554, 0.9238795325112850731, 1.000000000000000000, 0.9238795325112867385, 1.000000000000000000, 0.9238795325112867385, 1.000000000000000000, 0.9238795325112850731, 1.000000000000001554 ) ) 
 REPRESENTATION_ITEM ( '' )  );
#26859=CARTESIAN_POINT ( 'NONE',  ( -8.049105076161786076E-16, 34.99726562608393721, -13.14518615778179544 ) ) ;
#26864=CARTESIAN_POINT ( 'NONE',  ( 5.444914386472297529, 34.15390625108393863, -13.14518615778179722 ) ) ;
#26867=CARTESIAN_POINT ( 'NONE',  ( -5.622872871577920151, 36.38632812499999858, 13.57481594606300135 ) ) ;
#26871=CARTESIAN_POINT ( 'NONE',  ( 13.57481594606304576, 35.04687499999999289, -1.662435489736055892E-15 ) ) ;
#26872=CARTESIAN_POINT ( 'NONE',  ( 5.444914386472302859, 35.24531250108393010, 13.14518615778179189 ) ) ;
#26875=CARTESIAN_POINT ( 'NONE',  ( 6.944423797152706079, 31.55306878032414986, -11.16113333171310451 ) ) ;
#26905=CARTESIAN_POINT ( 'NONE',  ( -13.14518615778179544, 34.40195312608393152, 0.000000000000000000 ) ) ;
#26906=CARTESIAN_POINT ( 'NONE',  ( -9.598844408820458085, 34.65000000216787868, -9.598844408820458085 ) ) ;
#26929=CARTESIAN_POINT ( 'NONE',  ( -13.14518615778179900, 34.15390625108393863, -5.444914386472297529 ) ) ;
#26930=CARTESIAN_POINT ( 'NONE',  ( -8.312177448680279460E-16, 33.75703125216787726, -13.57481594606304576 ) ) ;
#26959=CARTESIAN_POINT ( 'NONE',  ( -13.14518615778179544, 33.40976562608393863, 0.000000000000000000 ) ) ;
#26978=CARTESIAN_POINT ( 'NONE',  ( 13.57481594606304576, 39.90859375216787441, -1.662435489736055892E-15 ) ) ;
#26998=CARTESIAN_POINT ( 'NONE',  ( -13.14518615778179544, 35.98945312608393721, 0.000000000000000000 ) ) ;
#27005=CARTESIAN_POINT ( 'NONE',  ( 9.295050272127046043, 34.10429687608393579, -9.295050272127046043 ) ) ;
#27011=CARTESIAN_POINT ( 'NONE',  ( 5.622872871577871301, 32.81445312499999289, -13.57481594606304753 ) ) ;
#27012=CARTESIAN_POINT ( 'NONE',  ( -13.14518615778179544, 34.99726562608393721, 0.000000000000000000 ) ) ;
#27046=CARTESIAN_POINT ( 'NONE',  ( 2.414731522848535132E-15, 33.80664062608393294, 13.14518615778179544 ) ) ;
#27047=CARTESIAN_POINT ( 'NONE',  ( 13.57481594606304753, 32.81445312716787299, -5.622872871577873077 ) ) ;
#27054=CARTESIAN_POINT ( 'NONE',  ( 2.493653234604083739E-15, 36.53515625216787299, 13.57481594606304576 ) ) ;
#27055=PRODUCT_DEFINITION ( 'UNKNOWN', '', #19955, #3511 ) ;
#27069=CARTESIAN_POINT ( 'NONE',  ( 9.295050272127047819, 33.70742187608393436, 9.295050272127046043 ) ) ;
#27076=FACE_OUTER_BOUND ( 'NONE', #21524, .T. ) ;
#27090=DIRECTION ( 'NONE',  ( -0.000000000000000000, -1.000000000000000000, -0.000000000000000000 ) ) ;
#27098=CARTESIAN_POINT ( 'NONE',  ( 2.414731522848535132E-15, 33.60820312608392868, 13.14518615778179544 ) ) ;
#27107=CARTESIAN_POINT ( 'NONE',  ( 13.57481594606304576, 35.93984375216787441, -1.662435489736055892E-15 ) ) ;
#27142=CARTESIAN_POINT ( 'NONE',  ( 5.622872871577928144, 38.46992187716787726, -13.57481594606299247 ) ) ;
#27143=CARTESIAN_POINT ( 'NONE',  ( -13.14518615778179544, 36.78320312608393294, 0.000000000000000000 ) ) ;
#27151=CARTESIAN_POINT ( 'NONE',  ( 9.295050272127047819, 33.90585937608393863, 9.295050272127046043 ) ) ;
#27156=CARTESIAN_POINT ( 'NONE',  ( -5.622872871577873077, 34.00507812499999716, 13.57481594606304753 ) ) ;
#27157=CARTESIAN_POINT ( 'NONE',  ( -9.295050272127046043, 34.10429687608393579, -9.295050272127046043 ) ) ;
#27167=CARTESIAN_POINT ( 'NONE',  ( -13.57481594606304398, 33.90585937499999858, 5.622872871577880183 ) ) ;
#27192=CARTESIAN_POINT ( 'NONE',  ( -5.444914386472297529, 34.25312500108393010, -13.14518615778179900 ) ) ;
#27193=CARTESIAN_POINT ( 'NONE',  ( 9.598844408820456309, 34.45156250216787441, -9.598844408820458085 ) ) ;
#27212=CARTESIAN_POINT ( 'NONE',  ( 9.295050272127047819, 32.11992187608393579, 9.295050272127046043 ) ) ;
#27234=ORIENTED_EDGE ( 'NONE', *, *, #8452, .T. ) ;
#27263=VERTEX_POINT ( 'NONE', #16671 ) ;
#27270=CARTESIAN_POINT ( 'NONE',  ( 2.414731522848535132E-15, 39.16445312608392726, 13.14518615778179544 ) ) ;
#27279=CARTESIAN_POINT ( 'NONE',  ( -13.14518615778179544, 33.60820312608393579, 0.000000000000000000 ) ) ;
#27285=CARTESIAN_POINT ( 'NONE',  ( -13.14518615778179189, 34.45156250108394147, 5.444914386472304635 ) ) ;
#27293=CARTESIAN_POINT ( 'NONE',  ( 5.444914386472302859, 32.07031250108393294, 13.14518615778179189 ) ) ;
#27304=EDGE_CURVE ( 'NONE', #15088, #11263, #15493, .T. ) ;
#27326=CARTESIAN_POINT ( 'NONE',  ( -9.598844408820454532, 38.71796874999999716, 9.598844408820459861 ) ) ;
#27327=CARTESIAN_POINT ( 'NONE',  ( -13.57481594606304576, 32.36796875216787583, 0.000000000000000000 ) ) ;
#27351=CARTESIAN_POINT ( 'NONE',  ( -8.049105076161786076E-16, 31.62382812608393579, -13.14518615778179544 ) ) ;
#27405=CARTESIAN_POINT ( 'NONE',  ( -9.295050272127044266, 39.06523437608392868, 9.295050272127047819 ) ) ;
#27410=CARTESIAN_POINT ( 'NONE',  ( 13.14518615778179900, 32.36796875108393579, 5.444914386472293977 ) ) ;
#27415=CARTESIAN_POINT ( 'NONE',  ( -8.312177448680279460E-16, 39.31328125216787583, -13.57481594606304576 ) ) ;
#27416=ORIENTED_EDGE ( 'NONE', *, *, #11740, .F. ) ;
#27423=CARTESIAN_POINT ( 'NONE',  ( -13.14518615778179900, 31.77265625108393365, -5.444914386472297529 ) ) ;
#27428=EDGE_CURVE ( 'NONE', #138, #2116, #23921, .T. ) ;
#27444=CARTESIAN_POINT ( 'NONE',  ( -13.57481594606304753, 40.15664062499999432, -5.622872871577872189 ) ) ;
#27460=CARTESIAN_POINT ( 'NONE',  ( 13.57481594606304931, 38.96601562499999005, 5.622872871577869525 ) ) ;
#27461=CARTESIAN_POINT ( 'NONE',  ( 9.598844408820459861, 31.87187500216787228, 9.598844408820456309 ) ) ;
#27468=( BOUNDED_CURVE ( )  B_SPLINE_CURVE ( 2, ( #14252, #16545, #24958, #5443, #9706, #3722, #12384, #22973, #20830 ),
 .UNSPECIFIED., .F., .F. ) 
 B_SPLINE_CURVE_WITH_KNOTS ( ( 3, 2, 2, 2, 3 ),
 ( 0.1041666666666664909, 0.1145833333333332732, 0.1250000000000000833, 0.1354166666666668517, 0.1458333333333336757 ),
 .UNSPECIFIED. ) 
 CURVE ( )  GEOMETRIC_REPRESENTATION_ITEM ( )  RATIONAL_B_SPLINE_CURVE ( ( 1.000000000000001332, 0.9238795325112854062, 1.000000000000000000, 0.9238795325112867385, 1.000000000000000000, 0.9238795325112867385, 1.000000000000000000, 0.9238795325112842960, 1.000000000000002442 ) ) 
 REPRESENTATION_ITEM ( '' )  );
#27484=ORIENTED_EDGE ( 'NONE', *, *, #8613, .T. ) ;
#27501=CARTESIAN_POINT ( 'NONE',  ( 9.598844408820456309, 39.21406250216787015, -9.598844408820458085 ) ) ;
#27516=CARTESIAN_POINT ( 'NONE',  ( 6.944423442990538931, 31.61921458391298856, -11.16113355206744195 ) ) ;
#27521=CARTESIAN_POINT ( 'NONE',  ( 2.493653234604083739E-15, 35.64218749999999147, 13.57481594606304576 ) ) ;
#27558=CARTESIAN_POINT ( 'NONE',  ( 9.295050272127046043, 32.51679687608393721, -9.295050272127046043 ) ) ;
#27586=CARTESIAN_POINT ( 'NONE',  ( -8.049105076161786076E-16, 39.75976562608394005, -13.14518615778179544 ) ) ;
#27593=CARTESIAN_POINT ( 'NONE',  ( 13.57481594606304931, 40.55351562499998863, 5.622872871577869525 ) ) ;
#27594=CARTESIAN_POINT ( 'NONE',  ( -9.295050272127046043, 39.66054687608393436, -9.295050272127046043 ) ) ;
#27607=ORIENTED_EDGE ( 'NONE', *, *, #24837, .T. ) ;
#27618=CARTESIAN_POINT ( 'NONE',  ( -9.598844408820454532, 32.46718750216787441, 9.598844408820459861 ) ) ;
#27628=( BOUNDED_CURVE ( )  B_SPLINE_CURVE ( 2, ( #20576, #27142, #7594, #24985, #5466, #14135, #22856, #21414, #19267 ),
 .UNSPECIFIED., .F., .F. ) 
 B_SPLINE_CURVE_WITH_KNOTS ( ( 3, 2, 2, 2, 3 ),
 ( 0.1875000000000001388, 0.1979166666666667407, 0.2083333333333333703, 0.2187499999999999722, 0.2291666666666665741 ),
 .UNSPECIFIED. ) 
 CURVE ( )  GEOMETRIC_REPRESENTATION_ITEM ( )  RATIONAL_B_SPLINE_CURVE ( ( 0.9999999999999990008, 0.9238795325112877377, 1.000000000000000000, 0.9238795325112867385, 1.000000000000000000, 0.9238795325112867385, 1.000000000000000000, 0.9238795325112872936, 0.9999999999999994449 ) ) 
 REPRESENTATION_ITEM ( '' )  );
#27635=CARTESIAN_POINT ( 'NONE',  ( -9.295050272127044266, 40.05742187608393579, 9.295050272127047819 ) ) ;
#27654=CARTESIAN_POINT ( 'NONE',  ( -13.14518615778179544, 38.96601562608393721, 0.000000000000000000 ) ) ;
#27665=ORIENTED_EDGE ( 'NONE', *, *, #10172, .T. ) ;
#27679=CARTESIAN_POINT ( 'NONE',  ( -13.14518615778179544, 39.75976562608393294, 0.000000000000000000 ) ) ;
#27690=CARTESIAN_POINT ( 'NONE',  ( -13.14518615778179189, 33.65781250108393152, 5.444914386472304635 ) ) ;
#27696=CARTESIAN_POINT ( 'NONE',  ( 13.57481594606304753, 39.16445312716788152, -5.622872871577873966 ) ) ;
#27718=PLANE ( 'NONE',  #8687 ) ;
#27724=CARTESIAN_POINT ( 'NONE',  ( -5.622872871577947684, 40.05742187499998863, -13.57481594606297293 ) ) ;
#27727=CARTESIAN_POINT ( 'NONE',  ( 13.14518615778179544, 40.35507812608393863, -1.609821015232357215E-15 ) ) ;
#27734=CARTESIAN_POINT ( 'NONE',  ( -13.57481594606304576, 40.99999999999999289, 0.000000000000000000 ) ) ;
#27735=CARTESIAN_POINT ( 'NONE',  ( -13.57481594606304576, 31.57421875216786944, 0.000000000000000000 ) ) ;
#27746=VECTOR ( 'NONE', #12191, 1000.000000000000000 ) ;
#27772=CARTESIAN_POINT ( 'NONE',  ( 13.14518615778179544, 39.56132812608393579, -1.609821015232357215E-15 ) ) ;
#27791=CARTESIAN_POINT ( 'NONE',  ( 5.444914386472302859, 38.42031250108393436, 13.14518615778179189 ) ) ;
#27811=CARTESIAN_POINT ( 'NONE',  ( 1.662435489736055892E-15, 40.99999999999999289, 13.57481594606304576 ) ) ;
#27813=ORIENTED_EDGE ( 'NONE', *, *, #10987, .F. ) ;
#27821=CARTESIAN_POINT ( 'NONE',  ( -13.14518615778179722, 39.71015625108393010, -5.444914386472297529 ) ) ;
#27832=CARTESIAN_POINT ( 'NONE',  ( -13.14518615778179900, 31.97109375108393436, -5.444914386472297529 ) ) ;
#27848=CARTESIAN_POINT ( 'NONE',  ( 13.57481594606304931, 34.99726562500000426, 5.622872871577868636 ) ) ;
#27859=CARTESIAN_POINT ( 'NONE',  ( -13.14518615778179544, 33.40976562608393863, 0.000000000000000000 ) ) ;
#27870=CARTESIAN_POINT ( 'NONE',  ( -13.14518615778179544, 32.02070312608393010, 0.000000000000000000 ) ) ;
#27871=CARTESIAN_POINT ( 'NONE',  ( 3.878385410779738418, 31.34156310770110565, -13.57481594606304931 ) ) ;
#27909=FACE_OUTER_BOUND ( 'NONE', #16370, .T. ) ;
#27917=VECTOR ( 'NONE', #11611, 1000.000000000000000 ) ;
#27921=CARTESIAN_POINT ( 'NONE',  ( 2.493653234604083739E-15, 38.81718749999999574, 13.57481594606304576 ) ) ;
#27925=CARTESIAN_POINT ( 'NONE',  ( -8.312177448680279460E-16, 38.42031249999999432, -13.57481594606304576 ) ) ;
#27950=EDGE_CURVE ( 'NONE', #22274, #24795, #16633, .T. ) ;
#27955=CARTESIAN_POINT ( 'NONE',  ( -8.049105076161786076E-16, 37.18007812608393436, -13.14518615778179544 ) ) ;
#27964=EDGE_CURVE ( 'NONE', #637, #8989, #25326, .T. ) ;
#27979=CARTESIAN_POINT ( 'NONE',  ( -5.622872871577873966, 36.98164062716787015, -13.57481594606304753 ) ) ;
#27989=CYLINDRICAL_SURFACE ( 'NONE', #617, 15.57481594606304576 ) ;
#27998=CARTESIAN_POINT ( 'NONE',  ( -5.444914386472297529, 38.22187500108393010, -13.14518615778179900 ) ) ;
#28000=CARTESIAN_POINT ( 'NONE',  ( 13.57481594606304931, 38.17226562499999432, 5.622872871577868636 ) ) ;
#28003=CARTESIAN_POINT ( 'NONE',  ( -13.14518615778179189, 40.00781250108393294, 5.444914386472304635 ) ) ;
#28010=CARTESIAN_POINT ( 'NONE',  ( 13.57481594606304931, 36.58476562499999574, 5.622872871577869525 ) ) ;
#28011=CARTESIAN_POINT ( 'NONE',  ( -9.295050272127046043, 36.48554687608393721, -9.295050272127046043 ) ) ;
#28024=CARTESIAN_POINT ( 'NONE',  ( -8.312177448680279460E-16, 37.72578125216787726, -13.57481594606304576 ) ) ;
#28027=VERTEX_POINT ( 'NONE', #18774 ) ;
#28028=CARTESIAN_POINT ( 'NONE',  ( -5.622872871577804688, 37.18007812499999432, 13.57481594606311504 ) ) ;
#28048=CARTESIAN_POINT ( 'NONE',  ( 13.14518615778179544, 40.35507812608393863, -1.609821015232357215E-15 ) ) ;
#28058=LINE ( 'NONE', #261, #19287 ) ;
#28066=CARTESIAN_POINT ( 'NONE',  ( 5.444914386472297529, 37.92421875108392726, -13.14518615778179900 ) ) ;
#28094=CARTESIAN_POINT ( 'NONE',  ( -9.295050272127044266, 37.47773437608393010, 9.295050272127047819 ) ) ;
#28134=CARTESIAN_POINT ( 'NONE',  ( -5.444914386472297529, 39.01562500108394005, -13.14518615778179900 ) ) ;
#28140=CARTESIAN_POINT ( 'NONE',  ( -13.14518615778179544, 39.95820312608393010, 0.000000000000000000 ) ) ;
#28148=CARTESIAN_POINT ( 'NONE',  ( 5.622872871577871301, 37.57695312499998863, -13.57481594606304753 ) ) ;
#28149=CARTESIAN_POINT ( 'NONE',  ( 13.14518615778179900, 37.03125000108393294, -5.444914386472297529 ) ) ;
#28158=DIRECTION ( 'NONE',  ( -0.000000000000000000, -1.000000000000000000, -0.000000000000000000 ) ) ;
#28163=CARTESIAN_POINT ( 'NONE',  ( -13.57481594606304576, 34.64999999999999147, 0.000000000000000000 ) ) ;
#28166=CARTESIAN_POINT ( 'NONE',  ( 2.493653234604083739E-15, 36.53515625216787299, 13.57481594606304576 ) ) ;
#28173=CARTESIAN_POINT ( 'NONE',  ( -8.312177448680279460E-16, 32.86406249999999574, -13.57481594606304576 ) ) ;
#28182=EDGE_CURVE ( 'NONE', #13527, #19588, #18047, .T. ) ;
#28185=CARTESIAN_POINT ( 'NONE',  ( 2.414731522848535132E-15, 37.77539062608393294, 13.14518615778179544 ) ) ;
#28186=CARTESIAN_POINT ( 'NONE',  ( 9.598844408820456309, 36.83281250216787583, -9.598844408820458085 ) ) ;
ENDSEC;
END-ISO-10303-21;
